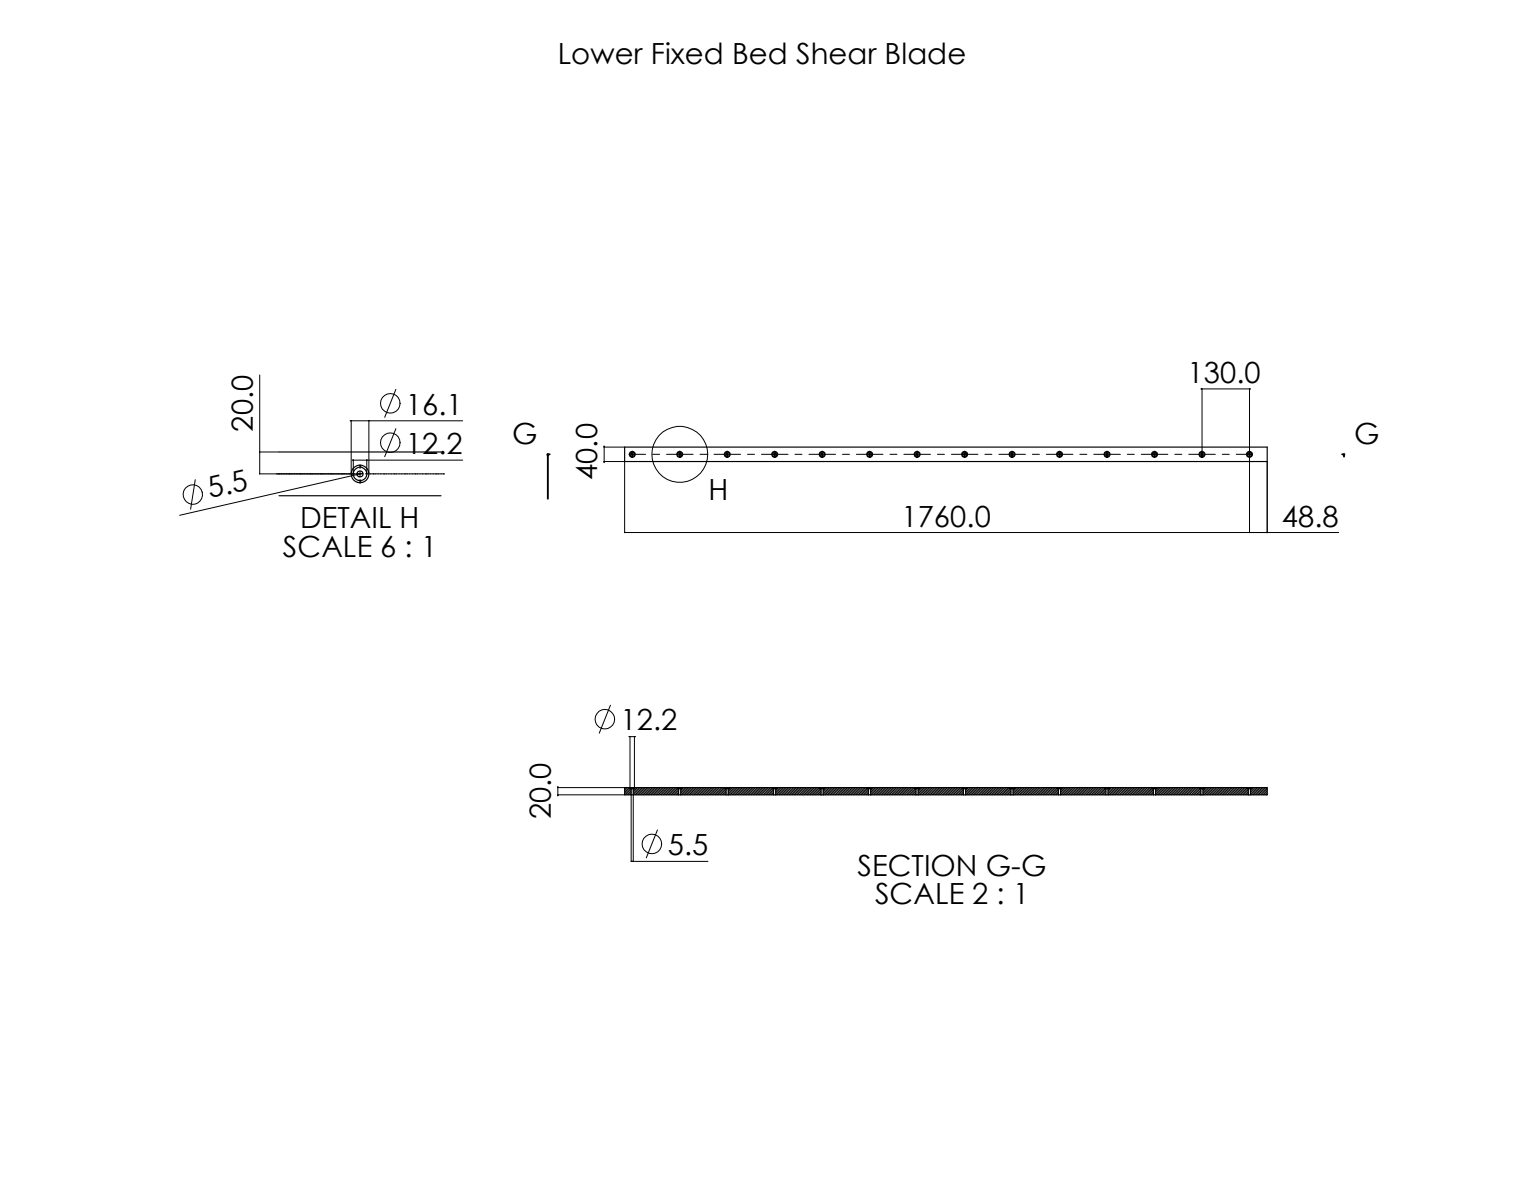
ISO-10303-21;
HEADER;
FILE_DESCRIPTION (('STEP AP214'),
    '1' );
FILE_NAME ('Lower Fixed Bed Shear Blade.step',
    '2026-10-21T17:07:05',
    ( '' ),
    ( '' ),
    'SwSTEP 2.0',
    'SolidWorks 2025',
    '' );
FILE_SCHEMA (( 'AUTOMOTIVE_DESIGN' ));
ENDSEC;

DATA;
#64=DIRECTION ( 'NONE',  ( 0.000000000000000000, 0.000000000000000000, 1.000000000000000000 ) ) ;
#90=EDGE_CURVE ( 'NONE', #25509, #42507, #33534, .T. ) ;
#102=FACE_OUTER_BOUND ( 'NONE', #34490, .T. ) ;
#109=EDGE_CURVE ( 'NONE', #28297, #10740, #37704, .T. ) ;
#136=CARTESIAN_POINT ( 'NONE',  ( 701.1634899080286232, 259.9999999999999432, -208.0249999999989825 ) ) ;
#150=CARTESIAN_POINT ( 'NONE',  ( 441.1634899080286232, 259.9999999999999432, -208.0249999999972488 ) ) ;
#156=CARTESIAN_POINT ( 'NONE',  ( 311.1634899080286232, 260.0000000000000000, -208.0249999999963109 ) ) ;
#168=CARTESIAN_POINT ( 'NONE',  ( -338.8365100919713200, 256.5000000000001137, -199.9999999999917861 ) ) ;
#175=ORIENTED_EDGE ( 'NONE', *, *, #22188, .T. ) ;
#215=DIRECTION ( 'NONE',  ( 0.000000000000000000, 0.000000000000000000, 1.000000000000000000 ) ) ;
#249=DIRECTION ( 'NONE',  ( -0.000000000000000000, 1.000000000000000000, -0.000000000000000000 ) ) ;
#252=ORIENTED_EDGE ( 'NONE', *, *, #2953, .T. ) ;
#299=ORIENTED_EDGE ( 'NONE', *, *, #28143, .F. ) ;
#323=CIRCLE ( 'NONE', #21716, 6.118999999999985562 ) ;
#329=AXIS2_PLACEMENT_3D ( 'NONE', #6576, #23655, #31056 ) ;
#334=PLANE ( 'NONE',  #18115 ) ;
#335=DIRECTION ( 'NONE',  ( -0.000000000000000000, 1.000000000000000000, -0.000000000000000000 ) ) ;
#344=CARTESIAN_POINT ( 'NONE',  ( 181.1634899080285948, 256.5000000000000000, -202.7499999999952820 ) ) ;
#355=AXIS2_PLACEMENT_3D ( 'NONE', #23312, #5092, #16163 ) ;
#363=DIRECTION ( 'NONE',  ( 0.000000000000000000, 0.000000000000000000, 1.000000000000000000 ) ) ;
#364=CARTESIAN_POINT ( 'NONE',  ( -202.7175100919714055, 256.5000000000001137, -199.9999999999926956 ) ) ;
#373=DIRECTION ( 'NONE',  ( 0.000000000000000000, 0.000000000000000000, 1.000000000000000000 ) ) ;
#391=CYLINDRICAL_SURFACE ( 'NONE', #1235, 2.749999999999863665 ) ;
#409=EDGE_CURVE ( 'NONE', #40245, #10694, #7775, .T. ) ;
#413=ORIENTED_EDGE ( 'NONE', *, *, #14771, .T. ) ;
#431=EDGE_CURVE ( 'NONE', #22786, #36028, #26937, .T. ) ;
#433=CARTESIAN_POINT ( 'NONE',  ( -78.83651009197140525, 240.0000000000000568, -199.9999999999936051 ) ) ;
#438=ORIENTED_EDGE ( 'NONE', *, *, #28628, .T. ) ;
#442=CARTESIAN_POINT ( 'NONE',  ( -852.7175100919713486, 256.5000000000002274, -199.9999999999881481 ) ) ;
#446=DIRECTION ( 'NONE',  ( -0.000000000000000000, 1.000000000000000000, -0.000000000000000000 ) ) ;
#448=VECTOR ( 'NONE', #36830, 999.9999999999998863 ) ;
#457=ADVANCED_FACE ( 'NONE', ( #28210 ), #41866, .F. ) ;
#466=VECTOR ( 'NONE', #30929, 1000.000000000000000 ) ;
#470=CARTESIAN_POINT ( 'NONE',  ( 831.1634899080286232, 259.9999999999998863, -199.9999999999999432 ) ) ;
#485=DIRECTION ( 'NONE',  ( -0.000000000000000000, 1.000000000000000000, -0.000000000000000000 ) ) ;
#490=AXIS2_PLACEMENT_3D ( 'NONE', #32758, #32530, #29065 ) ;
#509=DIRECTION ( 'NONE',  ( 0.000000000000000000, -1.000000000000000000, 0.000000000000000000 ) ) ;
#516=VECTOR ( 'NONE', #12520, 1000.000000000000000 ) ;
#521=EDGE_CURVE ( 'NONE', #12460, #20164, #17350, .T. ) ;
#527=ORIENTED_EDGE ( 'NONE', *, *, #24678, .F. ) ;
#530=ORIENTED_EDGE ( 'NONE', *, *, #3202, .F. ) ;
#547=CARTESIAN_POINT ( 'NONE',  ( 311.1634899080286232, 260.0000000000000000, -199.9999999999963336 ) ) ;
#567=CARTESIAN_POINT ( 'NONE',  ( 441.1634899080286232, 256.4999999999999432, -206.1189999999972144 ) ) ;
#569=EDGE_CURVE ( 'NONE', #23226, #12347, #33564, .T. ) ;
#599=LINE ( 'NONE', #35460, #21044 ) ;
#622=ADVANCED_FACE ( 'NONE', ( #10912, #13916, #35146, #24509, #31678, #3282, #39091, #20817, #34470, #34916, #6977, #31002, #31460, #31226, #3523 ), #24054, .F. ) ;
#663=CARTESIAN_POINT ( 'NONE',  ( -208.8365100919714052, 256.5000000000001137, -206.1189999999926954 ) ) ;
#664=DIRECTION ( 'NONE',  ( -0.000000000000000000, 1.000000000000000000, -0.000000000000000000 ) ) ;
#668=ORIENTED_EDGE ( 'NONE', *, *, #5793, .T. ) ;
#675=ADVANCED_FACE ( 'NONE', ( #20599 ), #14394, .F. ) ;
#678=CARTESIAN_POINT ( 'NONE',  ( 441.1634899080286232, 259.9999999999999432, -199.9999999999972431 ) ) ;
#682=DIRECTION ( 'NONE',  ( -0.000000000000000000, 1.000000000000000000, -0.000000000000000000 ) ) ;
#701=ORIENTED_EDGE ( 'NONE', *, *, #28035, .F. ) ;
#714=CARTESIAN_POINT ( 'NONE',  ( -78.83651009197140525, 256.5000000000000568, -202.7499999999934914 ) ) ;
#715=EDGE_CURVE ( 'NONE', #2952, #17860, #21035, .T. ) ;
#724=CARTESIAN_POINT ( 'NONE',  ( 571.1634899080285095, 259.9999999999999432, -199.9999999999981526 ) ) ;
#731=CARTESIAN_POINT ( 'NONE',  ( -208.8365100919714052, 258.0940000000001078, -193.8809999999926674 ) ) ;
#733=DIRECTION ( 'NONE',  ( -0.000000000000000000, 1.000000000000000000, -0.000000000000000000 ) ) ;
#746=ADVANCED_FACE ( 'NONE', ( #35841, #28910 ), #15052, .F. ) ;
#773=DIRECTION ( 'NONE',  ( 0.000000000000000000, 0.000000000000000000, 1.000000000000000000 ) ) ;
#774=ORIENTED_EDGE ( 'NONE', *, *, #715, .T. ) ;
#827=FACE_OUTER_BOUND ( 'NONE', #26973, .T. ) ;
#832=FACE_BOUND ( 'NONE', #35157, .T. ) ;
#873=CARTESIAN_POINT ( 'NONE',  ( -728.8365100919714905, 240.0000000000001990, -199.9999999999890861 ) ) ;
#891=DIRECTION ( 'NONE',  ( 0.000000000000000000, 0.000000000000000000, 1.000000000000000000 ) ) ;
#895=DIRECTION ( 'NONE',  ( 0.000000000000000000, 0.000000000000000000, 1.000000000000000000 ) ) ;
#910=DIRECTION ( 'NONE',  ( -0.000000000000000000, 1.000000000000000000, -0.000000000000000000 ) ) ;
#919=EDGE_CURVE ( 'NONE', #14904, #3234, #12181, .T. ) ;
#958=ORIENTED_EDGE ( 'NONE', *, *, #40695, .F. ) ;
#970=ADVANCED_FACE ( 'NONE', ( #44230 ), #9588, .F. ) ;
#973=ORIENTED_EDGE ( 'NONE', *, *, #27496, .F. ) ;
#980=AXIS2_PLACEMENT_3D ( 'NONE', #10116, #31353, #10336 ) ;
#996=CARTESIAN_POINT ( 'NONE',  ( -728.8365100919714905, 240.0000000000001990, -199.9999999999890861 ) ) ;
#1006=DIRECTION ( 'NONE',  ( -0.000000000000000000, 1.000000000000000000, -0.000000000000000000 ) ) ;
#1009=EDGE_CURVE ( 'NONE', #13600, #26360, #44455, .T. ) ;
#1018=ORIENTED_EDGE ( 'NONE', *, *, #15333, .T. ) ;
#1019=EDGE_CURVE ( 'NONE', #16583, #8247, #41590, .T. ) ;
#1047=CIRCLE ( 'NONE', #22428, 8.024999999999948841 ) ;
#1051=FACE_OUTER_BOUND ( 'NONE', #38699, .T. ) ;
#1054=FACE_BOUND ( 'NONE', #24359, .T. ) ;
#1074=ORIENTED_EDGE ( 'NONE', *, *, #6356, .T. ) ;
#1088=ORIENTED_EDGE ( 'NONE', *, *, #17337, .F. ) ;
#1099=CARTESIAN_POINT ( 'NONE',  ( 181.1634899080285948, 260.0000000000000000, -199.9999999999953957 ) ) ;
#1102=ORIENTED_EDGE ( 'NONE', *, *, #32866, .T. ) ;
#1119=CONICAL_SURFACE ( 'NONE', #17339, 8.024999999999948841, 0.7853981633974337351 ) ;
#1129=AXIS2_PLACEMENT_3D ( 'NONE', #37239, #8853, #9534 ) ;
#1134=CARTESIAN_POINT ( 'NONE',  ( 51.16348990802859475, 260.0000000000000568, -199.9999999999945146 ) ) ;
#1143=AXIS2_PLACEMENT_3D ( 'NONE', #37634, #44811, #30468 ) ;
#1174=AXIS2_PLACEMENT_3D ( 'NONE', #4069, #8002, #22282 ) ;
#1178=VECTOR ( 'NONE', #33127, 1000.000000000000114 ) ;
#1180=CARTESIAN_POINT ( 'NONE',  ( -468.8365100919714337, 256.5000000000001705, -202.7499999999907914 ) ) ;
#1201=ORIENTED_EDGE ( 'NONE', *, *, #10607, .T. ) ;
#1218=CARTESIAN_POINT ( 'NONE',  ( -728.8365100919714905, 260.0000000000001705, -199.9999999999890861 ) ) ;
#1235=AXIS2_PLACEMENT_3D ( 'NONE', #25558, #24866, #4321 ) ;
#1239=EDGE_CURVE ( 'NONE', #18073, #20679, #43780, .T. ) ;
#1246=VECTOR ( 'NONE', #42062, 1000.000000000000000 ) ;
#1251=ORIENTED_EDGE ( 'NONE', *, *, #3202, .T. ) ;
#1252=AXIS2_PLACEMENT_3D ( 'NONE', #35298, #45241, #3675 ) ;
#1269=ORIENTED_EDGE ( 'NONE', *, *, #27496, .T. ) ;
#1275=FACE_BOUND ( 'NONE', #36919, .T. ) ;
#1284=EDGE_CURVE ( 'NONE', #36701, #8042, #25367, .T. ) ;
#1288=CYLINDRICAL_SURFACE ( 'NONE', #20808, 2.749999999999863665 ) ;
#1322=ORIENTED_EDGE ( 'NONE', *, *, #35586, .F. ) ;
#1338=ADVANCED_FACE ( 'NONE', ( #17665 ), #34740, .F. ) ;
#1345=EDGE_LOOP ( 'NONE', ( #527, #16375 ) ) ;
#1364=DIRECTION ( 'NONE',  ( -0.000000000000000000, 1.000000000000000000, -0.000000000000000000 ) ) ;
#1383=ORIENTED_EDGE ( 'NONE', *, *, #22701, .F. ) ;
#1387=DIRECTION ( 'NONE',  ( -0.000000000000000000, 1.000000000000000000, -0.000000000000000000 ) ) ;
#1406=DIRECTION ( 'NONE',  ( 8.659560562354932858E-17, 0.7071067811865474617, -0.7071067811865474617 ) ) ;
#1432=ORIENTED_EDGE ( 'NONE', *, *, #25271, .T. ) ;
#1437=DIRECTION ( 'NONE',  ( 0.000000000000000000, 0.000000000000000000, 1.000000000000000000 ) ) ;
#1458=ORIENTED_EDGE ( 'NONE', *, *, #12287, .F. ) ;
#1471=ORIENTED_EDGE ( 'NONE', *, *, #8622, .T. ) ;
#1473=EDGE_LOOP ( 'NONE', ( #35327, #6545 ) ) ;
#1486=CARTESIAN_POINT ( 'NONE',  ( 441.1634899080286232, 259.9999999999999432, -199.9999999999972431 ) ) ;
#1521=EDGE_LOOP ( 'NONE', ( #973, #3985, #6124, #36419 ) ) ;
#1527=ORIENTED_EDGE ( 'NONE', *, *, #24375, .F. ) ;
#1572=ORIENTED_EDGE ( 'NONE', *, *, #41017, .T. ) ;
#1575=CYLINDRICAL_SURFACE ( 'NONE', #28444, 2.749999999999835687 ) ;
#1578=EDGE_CURVE ( 'NONE', #27745, #12435, #3971, .T. ) ;
#1584=DIRECTION ( 'NONE',  ( 0.000000000000000000, -1.000000000000000000, 0.000000000000000000 ) ) ;
#1614=DIRECTION ( 'NONE',  ( 0.000000000000000000, 0.000000000000000000, 1.000000000000000000 ) ) ;
#1671=DIRECTION ( 'NONE',  ( 1.892425610156518354E-16, 1.000000000000000000, -0.000000000000000000 ) ) ;
#1687=ORIENTED_EDGE ( 'NONE', *, *, #6335, .T. ) ;
#1730=CARTESIAN_POINT ( 'NONE',  ( 181.1634899080285948, 258.0939999999999941, -199.9999999999953957 ) ) ;
#1737=AXIS2_PLACEMENT_3D ( 'NONE', #29256, #18625, #39664 ) ;
#1789=EDGE_CURVE ( 'NONE', #18281, #21321, #6935, .T. ) ;
#1792=CARTESIAN_POINT ( 'NONE',  ( 181.1634899080285948, 258.0939999999999941, -193.8809999999953959 ) ) ;
#1821=DIRECTION ( 'NONE',  ( 8.659560562354884787E-17, 0.7071067811865513475, -0.7071067811865435759 ) ) ;
#1837=AXIS2_PLACEMENT_3D ( 'NONE', #10668, #24752, #17142 ) ;
#1841=AXIS2_PLACEMENT_3D ( 'NONE', #25140, #18248, #891 ) ;
#1848=EDGE_CURVE ( 'NONE', #24881, #7749, #17997, .T. ) ;
#1859=VECTOR ( 'NONE', #34701, 1000.000000000000000 ) ;
#1863=DIRECTION ( 'NONE',  ( 0.000000000000000000, 0.000000000000000000, 1.000000000000000000 ) ) ;
#1883=FACE_OUTER_BOUND ( 'NONE', #18472, .T. ) ;
#1903=CARTESIAN_POINT ( 'NONE',  ( 51.16348990802859475, 260.0000000000000568, -191.9749999999945089 ) ) ;
#1912=EDGE_LOOP ( 'NONE', ( #2855, #11798 ) ) ;
#1929=EDGE_LOOP ( 'NONE', ( #4719, #16342 ) ) ;
#1936=CARTESIAN_POINT ( 'NONE',  ( 571.1634899080285095, 259.9999999999999432, -191.9749999999982037 ) ) ;
#1953=AXIS2_PLACEMENT_3D ( 'NONE', #25021, #7703, #5081 ) ;
#1967=DIRECTION ( 'NONE',  ( -0.000000000000000000, 1.000000000000000000, -0.000000000000000000 ) ) ;
#1971=DIRECTION ( 'NONE',  ( 0.000000000000000000, 0.000000000000000000, 1.000000000000000000 ) ) ;
#2015=DIRECTION ( 'NONE',  ( 1.892425610156518354E-16, 1.000000000000000000, -0.000000000000000000 ) ) ;
#2021=ORIENTED_EDGE ( 'NONE', *, *, #18268, .F. ) ;
#2032=LINE ( 'NONE', #16126, #38083 ) ;
#2040=FACE_OUTER_BOUND ( 'NONE', #4448, .T. ) ;
#2052=ORIENTED_EDGE ( 'NONE', *, *, #41702, .T. ) ;
#2060=CARTESIAN_POINT ( 'NONE',  ( 51.16348990802859475, 260.0000000000000568, -208.0249999999945203 ) ) ;
#2071=DIRECTION ( 'NONE',  ( -0.000000000000000000, 1.000000000000000000, -0.000000000000000000 ) ) ;
#2089=DIRECTION ( 'NONE',  ( -1.000000000000000000, 0.000000000000000000, 0.000000000000000000 ) ) ;
#2109=ORIENTED_EDGE ( 'NONE', *, *, #27219, .T. ) ;
#2117=EDGE_CURVE ( 'NONE', #32983, #10586, #6970, .T. ) ;
#2155=AXIS2_PLACEMENT_3D ( 'NONE', #9924, #17090, #45047 ) ;
#2174=FACE_OUTER_BOUND ( 'NONE', #8874, .T. ) ;
#2183=DIRECTION ( 'NONE',  ( 0.000000000000000000, 0.000000000000000000, 1.000000000000000000 ) ) ;
#2184=DIRECTION ( 'NONE',  ( 0.000000000000000000, 0.000000000000000000, 1.000000000000000000 ) ) ;
#2187=DIRECTION ( 'NONE',  ( 1.892425610156518354E-16, 1.000000000000000000, -0.000000000000000000 ) ) ;
#2204=VERTEX_POINT ( 'NONE', #42077 ) ;
#2318=EDGE_LOOP ( 'NONE', ( #31488, #3719, #20337, #11430 ) ) ;
#2344=AXIS2_PLACEMENT_3D ( 'NONE', #37289, #19743, #2183 ) ;
#2350=DIRECTION ( 'NONE',  ( -0.000000000000000000, 1.000000000000000000, -0.000000000000000000 ) ) ;
#2371=AXIS2_PLACEMENT_3D ( 'NONE', #8273, #12193, #22338 ) ;
#2376=ORIENTED_EDGE ( 'NONE', *, *, #18681, .F. ) ;
#2429=ORIENTED_EDGE ( 'NONE', *, *, #24599, .T. ) ;
#2436=ORIENTED_EDGE ( 'NONE', *, *, #569, .F. ) ;
#2452=CYLINDRICAL_SURFACE ( 'NONE', #33609, 2.749999999999835687 ) ;
#2458=CIRCLE ( 'NONE', #980, 2.749999999999919176 ) ;
#2459=CARTESIAN_POINT ( 'NONE',  ( -598.8365100919716042, 256.5000000000001705, -193.8809999999899674 ) ) ;
#2469=CYLINDRICAL_SURFACE ( 'NONE', #21640, 2.749999999999835687 ) ;
#2489=ORIENTED_EDGE ( 'NONE', *, *, #9146, .F. ) ;
#2496=ORIENTED_EDGE ( 'NONE', *, *, #15984, .F. ) ;
#2521=VECTOR ( 'NONE', #28121, 1000.000000000000000 ) ;
#2523=CARTESIAN_POINT ( 'NONE',  ( -858.8365100919713768, 260.0000000000002274, -202.7499999999880345 ) ) ;
#2534=CARTESIAN_POINT ( 'NONE',  ( 571.1634899080285095, 256.4999999999999432, -199.9999999999981526 ) ) ;
#2538=VECTOR ( 'NONE', #9306, 1000.000000000000114 ) ;
#2565=VERTEX_POINT ( 'NONE', #39304 ) ;
#2570=AXIS2_PLACEMENT_3D ( 'NONE', #24286, #41626, #38393 ) ;
#2573=EDGE_LOOP ( 'NONE', ( #31065, #5375, #41524, #11084 ) ) ;
#2578=CIRCLE ( 'NONE', #34293, 2.749999999999842792 ) ;
#2586=VECTOR ( 'NONE', #42191, 1000.000000000000000 ) ;
#2621=EDGE_LOOP ( 'NONE', ( #6438, #44076, #22778, #12903 ) ) ;
#2629=AXIS2_PLACEMENT_3D ( 'NONE', #21604, #35686, #25291 ) ;
#2650=CARTESIAN_POINT ( 'NONE',  ( -338.8365100919713200, 240.0000000000001137, -199.9999999999917861 ) ) ;
#2665=DIRECTION ( 'NONE',  ( 0.000000000000000000, -1.000000000000000000, 0.000000000000000000 ) ) ;
#2691=AXIS2_PLACEMENT_3D ( 'NONE', #6556, #20411, #34260 ) ;
#2695=ADVANCED_FACE ( 'NONE', ( #18302 ), #32380, .F. ) ;
#2701=LINE ( 'NONE', #16798, #7052 ) ;
#2704=CARTESIAN_POINT ( 'NONE',  ( 571.1634899080285095, 256.4999999999999432, -199.9999999999981526 ) ) ;
#2718=MANIFOLD_SOLID_BREP ( 'CBORE for M5 Hex Head Bolt1[2]', #11423 ) ;
#2728=ORIENTED_EDGE ( 'NONE', *, *, #6661, .F. ) ;
#2736=VERTEX_POINT ( 'NONE', #44578 ) ;
#2744=EDGE_CURVE ( 'NONE', #13947, #12019, #37222, .T. ) ;
#2755=CARTESIAN_POINT ( 'NONE',  ( -879.9999999999992042, 260.0000000000002274, -219.9999999999999716 ) ) ;
#2758=CARTESIAN_POINT ( 'NONE',  ( -468.8365100919714337, 256.5000000000001705, -193.8809999999909053 ) ) ;
#2759=EDGE_CURVE ( 'NONE', #17388, #33219, #5502, .T. ) ;
#2800=AXIS2_PLACEMENT_3D ( 'NONE', #39327, #7928, #21531 ) ;
#2822=CARTESIAN_POINT ( 'NONE',  ( -858.8365100919713768, 256.5000000000002274, -193.8809999999881768 ) ) ;
#2855=ORIENTED_EDGE ( 'NONE', *, *, #19344, .F. ) ;
#2860=DIRECTION ( 'NONE',  ( -0.000000000000000000, 1.000000000000000000, -0.000000000000000000 ) ) ;
#2874=LINE ( 'NONE', #13736, #20844 ) ;
#2894=PLANE ( 'NONE',  #39520 ) ;
#2930=EDGE_CURVE ( 'NONE', #29766, #7990, #23958, .T. ) ;
#2941=CARTESIAN_POINT ( 'NONE',  ( -879.9999999999992042, 260.0000000000002274, -179.9999999999999716 ) ) ;
#2952=VERTEX_POINT ( 'NONE', #44343 ) ;
#2953=EDGE_CURVE ( 'NONE', #7990, #29766, #45355, .T. ) ;
#2963=ORIENTED_EDGE ( 'NONE', *, *, #31104, .T. ) ;
#2980=EDGE_CURVE ( 'NONE', #44849, #11829, #23929, .T. ) ;
#3007=EDGE_CURVE ( 'NONE', #41246, #7001, #8498, .T. ) ;
#3035=EDGE_LOOP ( 'NONE', ( #21215, #32230 ) ) ;
#3037=DIRECTION ( 'NONE',  ( -0.000000000000000000, 1.000000000000000000, -0.000000000000000000 ) ) ;
#3044=LINE ( 'NONE', #38609, #24699 ) ;
#3052=DIRECTION ( 'NONE',  ( 0.000000000000000000, 0.000000000000000000, 1.000000000000000000 ) ) ;
#3068=DIRECTION ( 'NONE',  ( -1.000000000000000000, 0.000000000000000000, 0.000000000000000000 ) ) ;
#3137=CARTESIAN_POINT ( 'NONE',  ( -208.8365100919714052, 256.5000000000001137, -202.7499999999925819 ) ) ;
#3138=LINE ( 'NONE', #38714, #14438 ) ;
#3140=VERTEX_POINT ( 'NONE', #17553 ) ;
#3161=CARTESIAN_POINT ( 'NONE',  ( -468.8365100919714337, 240.0000000000001421, -202.7499999999907345 ) ) ;
#3182=DIRECTION ( 'NONE',  ( -1.000000000000000000, 1.892425610156518354E-16, -0.000000000000000000 ) ) ;
#3202=EDGE_CURVE ( 'NONE', #30680, #28948, #34290, .T. ) ;
#3205=VERTEX_POINT ( 'NONE', #45260 ) ;
#3234=VERTEX_POINT ( 'NONE', #24684 ) ;
#3282=FACE_BOUND ( 'NONE', #18764, .T. ) ;
#3290=CIRCLE ( 'NONE', #45331, 8.024999999999948841 ) ;
#3299=ORIENTED_EDGE ( 'NONE', *, *, #19907, .F. ) ;
#3302=ORIENTED_EDGE ( 'NONE', *, *, #40695, .T. ) ;
#3305=( NAMED_UNIT ( * ) PLANE_ANGLE_UNIT ( ) SI_UNIT ( $, .RADIAN. ) );
#3318=DIRECTION ( 'NONE',  ( -0.000000000000000000, 1.000000000000000000, -0.000000000000000000 ) ) ;
#3323=DIRECTION ( 'NONE',  ( 0.000000000000000000, 0.000000000000000000, 1.000000000000000000 ) ) ;
#3327=CIRCLE ( 'NONE', #20980, 6.118999999999985562 ) ;
#3329=VECTOR ( 'NONE', #38752, 999.9999999999998863 ) ;
#3334=CARTESIAN_POINT ( 'NONE',  ( -728.8365100919714905, 260.0000000000001705, -208.0249999999890349 ) ) ;
#3336=CIRCLE ( 'NONE', #30589, 2.749999999999919176 ) ;
#3352=AXIS2_PLACEMENT_3D ( 'NONE', #10849, #17778, #32078 ) ;
#3356=DIRECTION ( 'NONE',  ( 0.000000000000000000, 0.000000000000000000, 1.000000000000000000 ) ) ;
#3357=CARTESIAN_POINT ( 'NONE',  ( -722.7175100919714623, 256.5000000000001705, -199.9999999999890861 ) ) ;
#3373=AXIS2_PLACEMENT_3D ( 'NONE', #20882, #23659, #3356 ) ;
#3388=EDGE_CURVE ( 'NONE', #10815, #22607, #39504, .T. ) ;
#3391=VECTOR ( 'NONE', #32469, 999.9999999999998863 ) ;
#3439=EDGE_LOOP ( 'NONE', ( #17422, #16149, #26248, #25911 ) ) ;
#3441=CARTESIAN_POINT ( 'NONE',  ( 831.1634899080286232, 256.4999999999998863, -197.2500000000000284 ) ) ;
#3443=CARTESIAN_POINT ( 'NONE',  ( -858.8365100919713768, 258.0940000000002215, -193.8809999999881768 ) ) ;
#3461=CIRCLE ( 'NONE', #25583, 6.118999999999985562 ) ;
#3488=EDGE_CURVE ( 'NONE', #26915, #40829, #16634, .T. ) ;
#3494=EDGE_LOOP ( 'NONE', ( #1018, #39594 ) ) ;
#3500=AXIS2_PLACEMENT_3D ( 'NONE', #44971, #38722, #41966 ) ;
#3510=ADVANCED_FACE ( 'NONE', ( #3911 ), #28380, .F. ) ;
#3523=FACE_OUTER_BOUND ( 'NONE', #33807, .T. ) ;
#3549=EDGE_CURVE ( 'NONE', #39281, #38048, #37255, .T. ) ;
#3560=CARTESIAN_POINT ( 'NONE',  ( -598.8365100919716042, 260.0000000000001705, -199.9999999999899671 ) ) ;
#3562=ORIENTED_EDGE ( 'NONE', *, *, #17880, .T. ) ;
#3569=AXIS2_PLACEMENT_3D ( 'NONE', #27047, #27953, #42049 ) ;
#3586=CARTESIAN_POINT ( 'NONE',  ( 701.1634899080286232, 259.9999999999999432, -199.9999999999990337 ) ) ;
#3617=FACE_OUTER_BOUND ( 'NONE', #40533, .T. ) ;
#3636=VECTOR ( 'NONE', #9011, 1000.000000000000114 ) ;
#3659=ORIENTED_EDGE ( 'NONE', *, *, #40850, .T. ) ;
#3662=EDGE_LOOP ( 'NONE', ( #22676, #3827, #31750, #2963 ) ) ;
#3675=DIRECTION ( 'NONE',  ( -1.000000000000000000, 0.000000000000000000, 0.000000000000000000 ) ) ;
#3679=CARTESIAN_POINT ( 'NONE',  ( -728.8365100919714905, 260.0000000000001705, -206.1189999999890574 ) ) ;
#3719=ORIENTED_EDGE ( 'NONE', *, *, #24375, .T. ) ;
#3721=DIRECTION ( 'NONE',  ( -0.000000000000000000, 1.000000000000000000, -0.000000000000000000 ) ) ;
#3774=DIRECTION ( 'NONE',  ( 0.000000000000000000, 0.000000000000000000, 1.000000000000000000 ) ) ;
#3775=CYLINDRICAL_SURFACE ( 'NONE', #33686, 2.749999999999863665 ) ;
#3787=DIRECTION ( 'NONE',  ( 0.000000000000000000, -0.000000000000000000, -1.000000000000000000 ) ) ;
#3827=ORIENTED_EDGE ( 'NONE', *, *, #13072, .F. ) ;
#3833=DIRECTION ( 'NONE',  ( 0.000000000000000000, 0.000000000000000000, 1.000000000000000000 ) ) ;
#3841=CARTESIAN_POINT ( 'NONE',  ( 51.16348990802859475, 260.0000000000000568, -199.9999999999945146 ) ) ;
#3842=EDGE_CURVE ( 'NONE', #40829, #26915, #24728, .T. ) ;
#3844=CYLINDRICAL_SURFACE ( 'NONE', #12912, 6.118999999999985562 ) ;
#3847=CARTESIAN_POINT ( 'NONE',  ( -858.8365100919713768, 256.5000000000002274, -199.9999999999881481 ) ) ;
#3858=ADVANCED_FACE ( 'NONE', ( #28917 ), #29596, .F. ) ;
#3862=CIRCLE ( 'NONE', #2344, 6.118999999999985562 ) ;
#3898=FACE_OUTER_BOUND ( 'NONE', #20408, .T. ) ;
#3905=FACE_BOUND ( 'NONE', #1345, .T. ) ;
#3911=FACE_OUTER_BOUND ( 'NONE', #37370, .T. ) ;
#3948=EDGE_LOOP ( 'NONE', ( #23305, #31638 ) ) ;
#3971=CIRCLE ( 'NONE', #15055, 2.749999999999919176 ) ;
#3978=ORIENTED_EDGE ( 'NONE', *, *, #6649, .F. ) ;
#3985=ORIENTED_EDGE ( 'NONE', *, *, #37858, .F. ) ;
#3992=ORIENTED_EDGE ( 'NONE', *, *, #37651, .F. ) ;
#4002=ORIENTED_EDGE ( 'NONE', *, *, #13445, .T. ) ;
#4007=ORIENTED_EDGE ( 'NONE', *, *, #13993, .F. ) ;
#4033=CARTESIAN_POINT ( 'NONE',  ( 879.9999999999992042, 259.9999999999998863, -219.9999999999999716 ) ) ;
#4052=EDGE_CURVE ( 'NONE', #40519, #28937, #18128, .T. ) ;
#4058=CIRCLE ( 'NONE', #19533, 2.749999999999919176 ) ;
#4062=CARTESIAN_POINT ( 'NONE',  ( 571.1634899080285095, 259.9999999999999432, -199.9999999999981526 ) ) ;
#4069=CARTESIAN_POINT ( 'NONE',  ( -468.8365100919714337, 256.5000000000001705, -199.9999999999908766 ) ) ;
#4087=CIRCLE ( 'NONE', #9970, 6.118999999999985562 ) ;
#4096=VECTOR ( 'NONE', #2071, 1000.000000000000000 ) ;
#4117=ORIENTED_EDGE ( 'NONE', *, *, #31446, .T. ) ;
#4128=EDGE_CURVE ( 'NONE', #29032, #40245, #25599, .T. ) ;
#4148=DIRECTION ( 'NONE',  ( 0.000000000000000000, -0.000000000000000000, -1.000000000000000000 ) ) ;
#4150=EDGE_CURVE ( 'NONE', #12347, #23226, #9248, .T. ) ;
#4168=AXIS2_PLACEMENT_3D ( 'NONE', #23038, #40839, #9199 ) ;
#4173=VECTOR ( 'NONE', #3721, 1000.000000000000000 ) ;
#4192=CARTESIAN_POINT ( 'NONE',  ( -728.8365100919714905, 240.0000000000001990, -197.2499999999891998 ) ) ;
#4216=DIRECTION ( 'NONE',  ( 0.000000000000000000, -0.000000000000000000, -1.000000000000000000 ) ) ;
#4237=ORIENTED_EDGE ( 'NONE', *, *, #5197, .T. ) ;
#4241=ORIENTED_EDGE ( 'NONE', *, *, #14801, .F. ) ;
#4249=CARTESIAN_POINT ( 'NONE',  ( 879.9999999999992042, 259.9999999999998863, -179.9999999999999716 ) ) ;
#4252=CARTESIAN_POINT ( 'NONE',  ( -858.8365100919713768, 260.0000000000002274, -199.9999999999881481 ) ) ;
#4276=DIRECTION ( 'NONE',  ( 0.000000000000000000, 0.000000000000000000, 1.000000000000000000 ) ) ;
#4302=CARTESIAN_POINT ( 'NONE',  ( 441.1634899080286232, 259.9999999999999432, -199.9999999999972431 ) ) ;
#4310=DIRECTION ( 'NONE',  ( 0.000000000000000000, 0.000000000000000000, 1.000000000000000000 ) ) ;
#4321=DIRECTION ( 'NONE',  ( 0.000000000000000000, 0.000000000000000000, 1.000000000000000000 ) ) ;
#4322=CARTESIAN_POINT ( 'NONE',  ( -468.8365100919714337, 256.5000000000001705, -206.1189999999908764 ) ) ;
#4328=DIRECTION ( 'NONE',  ( -0.000000000000000000, 1.000000000000000000, -0.000000000000000000 ) ) ;
#4338=ORIENTED_EDGE ( 'NONE', *, *, #32534, .F. ) ;
#4410=LINE ( 'NONE', #18501, #43969 ) ;
#4415=ORIENTED_EDGE ( 'NONE', *, *, #23048, .T. ) ;
#4423=DIRECTION ( 'NONE',  ( 8.659560562354807133E-17, 0.7071067811865578978, -0.7071067811865372477 ) ) ;
#4431=DIRECTION ( 'NONE',  ( -0.000000000000000000, 1.000000000000000000, -0.000000000000000000 ) ) ;
#4448=EDGE_LOOP ( 'NONE', ( #44211, #4584 ) ) ;
#4497=ORIENTED_EDGE ( 'NONE', *, *, #11378, .T. ) ;
#4510=VERTEX_POINT ( 'NONE', #4798 ) ;
#4524=CARTESIAN_POINT ( 'NONE',  ( 831.1634899080286232, 259.9999999999998863, -199.9999999999999432 ) ) ;
#4538=DIRECTION ( 'NONE',  ( -0.000000000000000000, 1.000000000000000000, -0.000000000000000000 ) ) ;
#4539=DIRECTION ( 'NONE',  ( -0.000000000000000000, 1.000000000000000000, -0.000000000000000000 ) ) ;
#4549=AXIS2_PLACEMENT_3D ( 'NONE', #35131, #31666, #20131 ) ;
#4555=ORIENTED_EDGE ( 'NONE', *, *, #16239, .T. ) ;
#4560=EDGE_LOOP ( 'NONE', ( #35172, #23960, #35397, #20708 ) ) ;
#4573=DIRECTION ( 'NONE',  ( -0.000000000000000000, 1.000000000000000000, -0.000000000000000000 ) ) ;
#4574=VERTEX_POINT ( 'NONE', #11956 ) ;
#4579=CARTESIAN_POINT ( 'NONE',  ( 441.1634899080286232, 259.9999999999999432, -191.9749999999972374 ) ) ;
#4584=ORIENTED_EDGE ( 'NONE', *, *, #17975, .T. ) ;
#4596=ORIENTED_EDGE ( 'NONE', *, *, #18756, .T. ) ;
#4600=CARTESIAN_POINT ( 'NONE',  ( -598.8365100919716042, 260.0000000000001705, -199.9999999999899671 ) ) ;
#4622=EDGE_CURVE ( 'NONE', #10881, #28279, #27703, .T. ) ;
#4629=VECTOR ( 'NONE', #39478, 1000.000000000000000 ) ;
#4662=DIRECTION ( 'NONE',  ( -0.000000000000000000, 1.000000000000000000, -0.000000000000000000 ) ) ;
#4663=ORIENTED_EDGE ( 'NONE', *, *, #37891, .T. ) ;
#4666=EDGE_CURVE ( 'NONE', #18328, #5387, #37183, .T. ) ;
#4670=ADVANCED_FACE ( 'NONE', ( #28490 ), #42807, .F. ) ;
#4707=DIRECTION ( 'NONE',  ( -0.000000000000000000, 1.000000000000000000, -0.000000000000000000 ) ) ;
#4719=ORIENTED_EDGE ( 'NONE', *, *, #26079, .F. ) ;
#4736=CARTESIAN_POINT ( 'NONE',  ( 441.1634899080286232, 259.9999999999999432, -199.9999999999972431 ) ) ;
#4744=DIRECTION ( 'NONE',  ( 0.000000000000000000, 0.000000000000000000, 1.000000000000000000 ) ) ;
#4748=CARTESIAN_POINT ( 'NONE',  ( 311.1634899080286232, 256.5000000000000000, -199.9999999999963336 ) ) ;
#4749=DIRECTION ( 'NONE',  ( 1.892425610156518354E-16, 1.000000000000000000, -0.000000000000000000 ) ) ;
#4760=CARTESIAN_POINT ( 'NONE',  ( -208.8365100919714052, 260.0000000000001137, -191.9749999999926899 ) ) ;
#4783=ORIENTED_EDGE ( 'NONE', *, *, #20154, .T. ) ;
#4797=AXIS2_PLACEMENT_3D ( 'NONE', #31895, #12938, #19635 ) ;
#4798=CARTESIAN_POINT ( 'NONE',  ( 571.1634899080285095, 256.4999999999999432, -202.7499999999980673 ) ) ;
#4816=AXIS2_PLACEMENT_3D ( 'NONE', #43754, #4978, #25975 ) ;
#4823=LINE ( 'NONE', #26048, #23213 ) ;
#4829=DIRECTION ( 'NONE',  ( 0.000000000000000000, 0.000000000000000000, 1.000000000000000000 ) ) ;
#4842=CIRCLE ( 'NONE', #2629, 8.025000000000003908 ) ;
#4845=APPLICATION_CONTEXT ( 'automotive_design' ) ;
#4865=CARTESIAN_POINT ( 'NONE',  ( 311.1634899080286232, 260.0000000000000000, -191.9749999999963279 ) ) ;
#4892=CARTESIAN_POINT ( 'NONE',  ( -78.83651009197140525, 240.0000000000000568, -199.9999999999936051 ) ) ;
#4909=DIRECTION ( 'NONE',  ( -1.000000000000000000, 0.000000000000000000, 0.000000000000000000 ) ) ;
#4910=DIRECTION ( 'NONE',  ( -0.000000000000000000, 1.000000000000000000, -0.000000000000000000 ) ) ;
#4917=CARTESIAN_POINT ( 'NONE',  ( 181.1634899080285948, 256.5000000000000000, -199.9999999999953957 ) ) ;
#4946=CIRCLE ( 'NONE', #1252, 2.749999999999863665 ) ;
#4947=ADVANCED_FACE ( 'NONE', ( #22451 ), #32643, .F. ) ;
#4968=DIRECTION ( 'NONE',  ( 0.000000000000000000, 0.7071067811865578978, 0.7071067811865372477 ) ) ;
#4971=PLANE ( 'NONE',  #8603 ) ;
#4978=DIRECTION ( 'NONE',  ( -0.000000000000000000, 1.000000000000000000, -0.000000000000000000 ) ) ;
#4981=CARTESIAN_POINT ( 'NONE',  ( 4.917854562272160638E-14, 260.0000000000000568, 0.000000000000000000 ) ) ;
#5042=VECTOR ( 'NONE', #10545, 1000.000000000000000 ) ;
#5052=CARTESIAN_POINT ( 'NONE',  ( 311.1634899080286232, 260.0000000000000000, -206.1189999999963050 ) ) ;
#5081=DIRECTION ( 'NONE',  ( 0.000000000000000000, 0.000000000000000000, 1.000000000000000000 ) ) ;
#5092=DIRECTION ( 'NONE',  ( -0.000000000000000000, 1.000000000000000000, -0.000000000000000000 ) ) ;
#5099=DIRECTION ( 'NONE',  ( 0.000000000000000000, 0.000000000000000000, 1.000000000000000000 ) ) ;
#5100=VECTOR ( 'NONE', #1406, 1000.000000000000114 ) ;
#5120=ORIENTED_EDGE ( 'NONE', *, *, #17979, .T. ) ;
#5128=EDGE_LOOP ( 'NONE', ( #31025, #26277, #29605, #7705 ) ) ;
#5155=CARTESIAN_POINT ( 'NONE',  ( -72.71751009197140547, 256.5000000000000568, -199.9999999999936051 ) ) ;
#5174=EDGE_LOOP ( 'NONE', ( #28986, #24546, #35045, #12721 ) ) ;
#5185=FACE_OUTER_BOUND ( 'NONE', #13079, .T. ) ;
#5191=DIRECTION ( 'NONE',  ( 0.000000000000000000, 0.000000000000000000, 1.000000000000000000 ) ) ;
#5194=FACE_BOUND ( 'NONE', #1912, .T. ) ;
#5197=EDGE_CURVE ( 'NONE', #44027, #33524, #21919, .T. ) ;
#5207=LINE ( 'NONE', #11707, #23915 ) ;
#5259=ORIENTED_EDGE ( 'NONE', *, *, #16521, .F. ) ;
#5280=EDGE_LOOP ( 'NONE', ( #30765, #27271, #4117, #12240 ) ) ;
#5298=VERTEX_POINT ( 'NONE', #12984 ) ;
#5311=CARTESIAN_POINT ( 'NONE',  ( 51.16348990802859475, 256.5000000000000568, -199.9999999999945146 ) ) ;
#5328=DIRECTION ( 'NONE',  ( -0.000000000000000000, 1.000000000000000000, -0.000000000000000000 ) ) ;
#5329=ORIENTED_EDGE ( 'NONE', *, *, #23218, .F. ) ;
#5346=DIRECTION ( 'NONE',  ( 0.000000000000000000, 0.000000000000000000, 1.000000000000000000 ) ) ;
#5347=CARTESIAN_POINT ( 'NONE',  ( 701.1634899080286232, 256.4999999999999432, -202.7499999999989484 ) ) ;
#5375=ORIENTED_EDGE ( 'NONE', *, *, #36816, .T. ) ;
#5383=VERTEX_POINT ( 'NONE', #5347 ) ;
#5387=VERTEX_POINT ( 'NONE', #40922 ) ;
#5410=EDGE_CURVE ( 'NONE', #26360, #5298, #6267, .T. ) ;
#5417=VECTOR ( 'NONE', #19310, 1000.000000000000000 ) ;
#5431=ADVANCED_FACE ( 'NONE', ( #1883 ), #20126, .F. ) ;
#5502=CIRCLE ( 'NONE', #32826, 6.119000000000013095 ) ;
#5549=CIRCLE ( 'NONE', #31374, 8.025000000000003908 ) ;
#5572=ORIENTED_EDGE ( 'NONE', *, *, #33916, .T. ) ;
#5580=AXIS2_PLACEMENT_3D ( 'NONE', #364, #36154, #21834 ) ;
#5582=FACE_OUTER_BOUND ( 'NONE', #12309, .T. ) ;
#5583=CARTESIAN_POINT ( 'NONE',  ( -338.8365100919713200, 260.0000000000001137, -199.9999999999917861 ) ) ;
#5589=CARTESIAN_POINT ( 'NONE',  ( -78.83651009197140525, 256.5000000000000568, -193.8809999999935769 ) ) ;
#5608=AXIS2_PLACEMENT_3D ( 'NONE', #20405, #2860, #45598 ) ;
#5613=AXIS2_PLACEMENT_3D ( 'NONE', #4302, #31997, #7762 ) ;
#5619=ORIENTED_EDGE ( 'NONE', *, *, #36478, .F. ) ;
#5621=AXIS2_PLACEMENT_3D ( 'NONE', #44533, #33682, #23273 ) ;
#5633=DIRECTION ( 'NONE',  ( -0.000000000000000000, 1.000000000000000000, -0.000000000000000000 ) ) ;
#5654=CIRCLE ( 'NONE', #490, 6.118999999999985562 ) ;
#5666=DIRECTION ( 'NONE',  ( 0.000000000000000000, 0.000000000000000000, 1.000000000000000000 ) ) ;
#5682=AXIS2_PLACEMENT_3D ( 'NONE', #26817, #30075, #9289 ) ;
#5689=EDGE_CURVE ( 'NONE', #2565, #32511, #24097, .T. ) ;
#5693=CIRCLE ( 'NONE', #14587, 6.118999999999985562 ) ;
#5700=DIRECTION ( 'NONE',  ( 0.000000000000000000, 0.000000000000000000, 1.000000000000000000 ) ) ;
#5714=EDGE_LOOP ( 'NONE', ( #28871, #23285, #1471, #25341 ) ) ;
#5757=ADVANCED_FACE ( 'NONE', ( #3905, #18000 ), #32070, .F. ) ;
#5761=ADVANCED_FACE ( 'NONE', ( #42925 ), #32540, .F. ) ;
#5764=ORIENTED_EDGE ( 'NONE', *, *, #17939, .F. ) ;
#5779=CARTESIAN_POINT ( 'NONE',  ( -598.8365100919716042, 258.0940000000001646, -199.9999999999899671 ) ) ;
#5793=EDGE_CURVE ( 'NONE', #8042, #36701, #13080, .T. ) ;
#5829=EDGE_CURVE ( 'NONE', #8740, #45067, #42592, .T. ) ;
#5888=CARTESIAN_POINT ( 'NONE',  ( 311.1634899080286232, 260.0000000000000000, -199.9999999999963336 ) ) ;
#5899=DIRECTION ( 'NONE',  ( -0.000000000000000000, 1.000000000000000000, -0.000000000000000000 ) ) ;
#5913=ORIENTED_EDGE ( 'NONE', *, *, #36558, .T. ) ;
#5920=LINE ( 'NONE', #40802, #26943 ) ;
#5971=ORIENTED_EDGE ( 'NONE', *, *, #43110, .F. ) ;
#5975=DIRECTION ( 'NONE',  ( -0.000000000000000000, 1.000000000000000000, -0.000000000000000000 ) ) ;
#6005=ORIENTED_EDGE ( 'NONE', *, *, #9679, .T. ) ;
#6014=LINE ( 'NONE', #16415, #10919 ) ;
#6020=EDGE_CURVE ( 'NONE', #14400, #22607, #32769, .T. ) ;
#6024=ORIENTED_EDGE ( 'NONE', *, *, #409, .T. ) ;
#6043=EDGE_CURVE ( 'NONE', #25919, #41246, #11529, .T. ) ;
#6059=LINE ( 'NONE', #13240, #1859 ) ;
#6075=DIRECTION ( 'NONE',  ( 1.000000000000000000, 0.000000000000000000, 0.000000000000000000 ) ) ;
#6089=DIRECTION ( 'NONE',  ( -0.000000000000000000, 1.000000000000000000, -0.000000000000000000 ) ) ;
#6092=CARTESIAN_POINT ( 'NONE',  ( 441.1634899080286232, 259.9999999999999432, -197.2499999999973852 ) ) ;
#6096=CARTESIAN_POINT ( 'NONE',  ( 831.1634899080286232, 259.9999999999998863, -199.9999999999999432 ) ) ;
#6120=EDGE_CURVE ( 'NONE', #28948, #42674, #8072, .T. ) ;
#6124=ORIENTED_EDGE ( 'NONE', *, *, #26419, .T. ) ;
#6145=DIRECTION ( 'NONE',  ( 0.000000000000000000, 0.000000000000000000, 1.000000000000000000 ) ) ;
#6153=CARTESIAN_POINT ( 'NONE',  ( -468.8365100919714337, 260.0000000000001705, -199.9999999999908766 ) ) ;
#6167=LINE ( 'NONE', #2941, #28653 ) ;
#6170=ORIENTED_EDGE ( 'NONE', *, *, #24477, .T. ) ;
#6267=LINE ( 'NONE', #30764, #516 ) ;
#6274=DIRECTION ( 'NONE',  ( -0.000000000000000000, 1.000000000000000000, -0.000000000000000000 ) ) ;
#6281=DIRECTION ( 'NONE',  ( 1.892425610156518354E-16, 1.000000000000000000, -0.000000000000000000 ) ) ;
#6288=CIRCLE ( 'NONE', #44636, 2.749999999999919176 ) ;
#6304=AXIS2_PLACEMENT_3D ( 'NONE', #873, #8267, #7828 ) ;
#6309=CIRCLE ( 'NONE', #32129, 2.749999999999919176 ) ;
#6323=FACE_OUTER_BOUND ( 'NONE', #17699, .T. ) ;
#6325=AXIS2_PLACEMENT_3D ( 'NONE', #14699, #17921, #363 ) ;
#6335=EDGE_CURVE ( 'NONE', #28948, #30680, #35859, .T. ) ;
#6343=DIRECTION ( 'NONE',  ( -0.000000000000000000, 1.000000000000000000, -0.000000000000000000 ) ) ;
#6353=CIRCLE ( 'NONE', #9935, 2.749999999999919176 ) ;
#6356=EDGE_CURVE ( 'NONE', #7990, #28297, #7271, .T. ) ;
#6357=FACE_OUTER_BOUND ( 'NONE', #38991, .T. ) ;
#6409=CYLINDRICAL_SURFACE ( 'NONE', #8359, 2.749999999999863665 ) ;
#6413=DIRECTION ( 'NONE',  ( -0.000000000000000000, 1.000000000000000000, -0.000000000000000000 ) ) ;
#6426=CIRCLE ( 'NONE', #36655, 2.749999999999835687 ) ;
#6436=CARTESIAN_POINT ( 'NONE',  ( -78.83651009197140525, 260.0000000000000568, -199.9999999999936051 ) ) ;
#6438=ORIENTED_EDGE ( 'NONE', *, *, #10590, .F. ) ;
#6506=CARTESIAN_POINT ( 'NONE',  ( 571.1634899080285095, 259.9999999999999432, -199.9999999999981526 ) ) ;
#6545=ORIENTED_EDGE ( 'NONE', *, *, #26084, .T. ) ;
#6556=CARTESIAN_POINT ( 'NONE',  ( 831.1634899080286232, 258.0939999999998804, -199.9999999999999432 ) ) ;
#6563=CARTESIAN_POINT ( 'NONE',  ( -208.8365100919714052, 260.0000000000001137, -199.9999999999926956 ) ) ;
#6576=CARTESIAN_POINT ( 'NONE',  ( -592.7175100919715760, 256.5000000000001705, -199.9999999999899671 ) ) ;
#6582=CARTESIAN_POINT ( 'NONE',  ( -858.8365100919713768, 256.5000000000002274, -202.7499999999880913 ) ) ;
#6583=FACE_OUTER_BOUND ( 'NONE', #27409, .T. ) ;
#6601=ORIENTED_EDGE ( 'NONE', *, *, #39633, .T. ) ;
#6649=EDGE_CURVE ( 'NONE', #20679, #40483, #8392, .T. ) ;
#6661=EDGE_CURVE ( 'NONE', #28937, #40519, #32165, .T. ) ;
#6698=ADVANCED_FACE ( 'NONE', ( #22461 ), #26260, .F. ) ;
#6706=CYLINDRICAL_SURFACE ( 'NONE', #3569, 6.118999999999985562 ) ;
#6742=DIRECTION ( 'NONE',  ( -0.000000000000000000, 1.000000000000000000, -0.000000000000000000 ) ) ;
#6770=ORIENTED_EDGE ( 'NONE', *, *, #17975, .F. ) ;
#6775=DIRECTION ( 'NONE',  ( -0.000000000000000000, 1.000000000000000000, -0.000000000000000000 ) ) ;
#6776=VERTEX_POINT ( 'NONE', #31948 ) ;
#6783=DIRECTION ( 'NONE',  ( -0.000000000000000000, 1.000000000000000000, -0.000000000000000000 ) ) ;
#6808=VERTEX_POINT ( 'NONE', #39829 ) ;
#6838=DIRECTION ( 'NONE',  ( -0.000000000000000000, 1.000000000000000000, -0.000000000000000000 ) ) ;
#6843=CARTESIAN_POINT ( 'NONE',  ( -879.9999999999992042, 260.0000000000002274, -219.9999999999999716 ) ) ;
#6859=LINE ( 'NONE', #34807, #3329 ) ;
#6861=ORIENTED_EDGE ( 'NONE', *, *, #44042, .T. ) ;
#6877=EDGE_LOOP ( 'NONE', ( #26194, #37083, #40389, #16437 ) ) ;
#6934=CARTESIAN_POINT ( 'NONE',  ( 831.1634899080286232, 239.9999999999998863, -202.7499999999998295 ) ) ;
#6935=CIRCLE ( 'NONE', #36445, 8.025000000000003908 ) ;
#6970=CIRCLE ( 'NONE', #34248, 2.749999999999835687 ) ;
#6977=FACE_BOUND ( 'NONE', #3494, .T. ) ;
#7001=VERTEX_POINT ( 'NONE', #9058 ) ;
#7018=AXIS2_PLACEMENT_3D ( 'NONE', #17935, #32004, #14477 ) ;
#7028=AXIS2_PLACEMENT_3D ( 'NONE', #19278, #29904, #43094 ) ;
#7033=DIRECTION ( 'NONE',  ( -0.000000000000000000, 1.000000000000000000, -0.000000000000000000 ) ) ;
#7041=AXIS2_PLACEMENT_3D ( 'NONE', #42304, #17833, #21063 ) ;
#7052=VECTOR ( 'NONE', #44972, 1000.000000000000000 ) ;
#7138=FACE_OUTER_BOUND ( 'NONE', #18912, .T. ) ;
#7146=ORIENTED_EDGE ( 'NONE', *, *, #14334, .T. ) ;
#7153=AXIS2_PLACEMENT_3D ( 'NONE', #17028, #31105, #13565 ) ;
#7167=CIRCLE ( 'NONE', #23358, 2.749999999999891642 ) ;
#7182=AXIS2_PLACEMENT_3D ( 'NONE', #28623, #31621, #42704 ) ;
#7193=LINE ( 'NONE', #35345, #4173 ) ;
#7196=DIRECTION ( 'NONE',  ( 0.000000000000000000, 0.7071067811865501263, 0.7071067811865449082 ) ) ;
#7197=EDGE_CURVE ( 'NONE', #40483, #21723, #6353, .T. ) ;
#7233=EDGE_LOOP ( 'NONE', ( #6601, #4596 ) ) ;
#7244=ORIENTED_EDGE ( 'NONE', *, *, #44042, .F. ) ;
#7265=DIRECTION ( 'NONE',  ( -0.000000000000000000, 1.000000000000000000, -0.000000000000000000 ) ) ;
#7271=LINE ( 'NONE', #31275, #25431 ) ;
#7285=DIRECTION ( 'NONE',  ( 0.000000000000000000, 0.000000000000000000, 1.000000000000000000 ) ) ;
#7289=ORIENTED_EDGE ( 'NONE', *, *, #5689, .T. ) ;
#7312=EDGE_LOOP ( 'NONE', ( #17467, #34606 ) ) ;
#7320=DIRECTION ( 'NONE',  ( 0.000000000000000000, 0.000000000000000000, 1.000000000000000000 ) ) ;
#7334=CARTESIAN_POINT ( 'NONE',  ( -728.8365100919714905, 260.0000000000001705, -199.9999999999890861 ) ) ;
#7352=AXIS2_PLACEMENT_3D ( 'NONE', #44672, #23628, #9568 ) ;
#7366=LINE ( 'NONE', #21217, #10792 ) ;
#7417=FACE_BOUND ( 'NONE', #11138, .T. ) ;
#7434=CARTESIAN_POINT ( 'NONE',  ( -468.8365100919714337, 260.0000000000001705, -199.9999999999908766 ) ) ;
#7456=ORIENTED_EDGE ( 'NONE', *, *, #3842, .T. ) ;
#7458=DIRECTION ( 'NONE',  ( -0.000000000000000000, 1.000000000000000000, -0.000000000000000000 ) ) ;
#7475=LINE ( 'NONE', #35627, #27014 ) ;
#7482=ORIENTED_EDGE ( 'NONE', *, *, #43367, .T. ) ;
#7489=DIRECTION ( 'NONE',  ( 0.000000000000000000, 0.000000000000000000, 1.000000000000000000 ) ) ;
#7492=CARTESIAN_POINT ( 'NONE',  ( -208.8365100919714052, 258.0940000000001078, -199.9999999999926956 ) ) ;
#7494=EDGE_CURVE ( 'NONE', #36773, #31071, #3044, .T. ) ;
#7505=DIRECTION ( 'NONE',  ( -1.000000000000000000, 1.880165489482579047E-16, 0.000000000000000000 ) ) ;
#7509=ORIENTED_EDGE ( 'NONE', *, *, #16501, .F. ) ;
#7523=ORIENTED_EDGE ( 'NONE', *, *, #23757, .F. ) ;
#7526=EDGE_LOOP ( 'NONE', ( #44778, #13250, #12647, #22491 ) ) ;
#7533=ORIENTED_EDGE ( 'NONE', *, *, #18143, .F. ) ;
#7550=EDGE_CURVE ( 'NONE', #10866, #11865, #2578, .T. ) ;
#7570=ORIENTED_EDGE ( 'NONE', *, *, #15389, .T. ) ;
#7627=VERTEX_POINT ( 'NONE', #2822 ) ;
#7640=LINE ( 'NONE', #8110, #14493 ) ;
#7644=ORIENTED_EDGE ( 'NONE', *, *, #43110, .T. ) ;
#7656=CARTESIAN_POINT ( 'NONE',  ( 181.1634899080285948, 260.0000000000000000, -191.9749999999953900 ) ) ;
#7698=DIRECTION ( 'NONE',  ( -0.000000000000000000, 1.000000000000000000, -0.000000000000000000 ) ) ;
#7699=ADVANCED_FACE ( 'NONE', ( #28680 ), #12905, .F. ) ;
#7702=DIRECTION ( 'NONE',  ( 0.000000000000000000, 0.000000000000000000, 1.000000000000000000 ) ) ;
#7703=DIRECTION ( 'NONE',  ( -0.000000000000000000, 1.000000000000000000, -0.000000000000000000 ) ) ;
#7705=ORIENTED_EDGE ( 'NONE', *, *, #25271, .F. ) ;
#7749=VERTEX_POINT ( 'NONE', #731 ) ;
#7759=AXIS2_PLACEMENT_3D ( 'NONE', #25766, #32479, #5191 ) ;
#7762=DIRECTION ( 'NONE',  ( 0.000000000000000000, 0.000000000000000000, 1.000000000000000000 ) ) ;
#7770=CARTESIAN_POINT ( 'NONE',  ( 571.1634899080285095, 259.9999999999999432, -199.9999999999981526 ) ) ;
#7771=PLANE ( 'NONE',  #45215 ) ;
#7775=CIRCLE ( 'NONE', #1129, 2.749999999999891642 ) ;
#7791=EDGE_CURVE ( 'NONE', #32511, #21321, #32136, .T. ) ;
#7799=AXIS2_PLACEMENT_3D ( 'NONE', #14200, #4707, #7285 ) ;
#7828=DIRECTION ( 'NONE',  ( -1.000000000000000000, 0.000000000000000000, 0.000000000000000000 ) ) ;
#7835=CARTESIAN_POINT ( 'NONE',  ( 311.1634899080286232, 260.0000000000000000, -199.9999999999963336 ) ) ;
#7864=AXIS2_PLACEMENT_3D ( 'NONE', #4600, #1364, #4829 ) ;
#7904=AXIS2_PLACEMENT_3D ( 'NONE', #6153, #34568, #20917 ) ;
#7908=( LENGTH_UNIT ( ) NAMED_UNIT ( * ) SI_UNIT ( .MILLI., .METRE. ) );
#7928=DIRECTION ( 'NONE',  ( 1.892425610156518354E-16, 1.000000000000000000, -0.000000000000000000 ) ) ;
#7946=DIRECTION ( 'NONE',  ( 0.000000000000000000, 0.000000000000000000, 1.000000000000000000 ) ) ;
#7962=VECTOR ( 'NONE', #5328, 1000.000000000000000 ) ;
#7990=VERTEX_POINT ( 'NONE', #12034 ) ;
#8000=ORIENTED_EDGE ( 'NONE', *, *, #13409, .T. ) ;
#8002=DIRECTION ( 'NONE',  ( -0.000000000000000000, 1.000000000000000000, -0.000000000000000000 ) ) ;
#8006=DIRECTION ( 'NONE',  ( -1.000000000000000000, 0.000000000000000000, 0.000000000000000000 ) ) ;
#8019=CARTESIAN_POINT ( 'NONE',  ( -78.83651009197140525, 260.0000000000000568, -197.2499999999937756 ) ) ;
#8024=AXIS2_PLACEMENT_3D ( 'NONE', #38580, #39271, #35106 ) ;
#8042=VERTEX_POINT ( 'NONE', #33945 ) ;
#8063=EDGE_CURVE ( 'NONE', #17707, #2736, #38007, .T. ) ;
#8069=ORIENTED_EDGE ( 'NONE', *, *, #17979, .F. ) ;
#8072=LINE ( 'NONE', #22134, #38911 ) ;
#8094=EDGE_CURVE ( 'NONE', #27562, #41260, #4087, .T. ) ;
#8110=CARTESIAN_POINT ( 'NONE',  ( -78.83651009197140525, 260.0000000000000568, -193.8809999999935769 ) ) ;
#8113=FACE_OUTER_BOUND ( 'NONE', #9283, .T. ) ;
#8148=LINE ( 'NONE', #35611, #28622 ) ;
#8149=VERTEX_POINT ( 'NONE', #41345 ) ;
#8158=EDGE_LOOP ( 'NONE', ( #11451, #39576, #33005, #25466 ) ) ;
#8217=DIRECTION ( 'NONE',  ( -0.000000000000000000, 1.000000000000000000, -0.000000000000000000 ) ) ;
#8232=LINE ( 'NONE', #25988, #31317 ) ;
#8247=VERTEX_POINT ( 'NONE', #20543 ) ;
#8267=DIRECTION ( 'NONE',  ( 1.892425610156518354E-16, 1.000000000000000000, -0.000000000000000000 ) ) ;
#8273=CARTESIAN_POINT ( 'NONE',  ( -208.8365100919714052, 260.0000000000001137, -199.9999999999926956 ) ) ;
#8288=ORIENTED_EDGE ( 'NONE', *, *, #43103, .T. ) ;
#8294=ORIENTED_EDGE ( 'NONE', *, *, #21009, .T. ) ;
#8297=DIRECTION ( 'NONE',  ( -0.000000000000000000, 1.000000000000000000, -0.000000000000000000 ) ) ;
#8315=ORIENTED_EDGE ( 'NONE', *, *, #4666, .T. ) ;
#8334=CARTESIAN_POINT ( 'NONE',  ( -728.8365100919714905, 256.5000000000001705, -193.8809999999890863 ) ) ;
#8359=AXIS2_PLACEMENT_3D ( 'NONE', #27637, #24392, #13562 ) ;
#8392=LINE ( 'NONE', #32654, #32058 ) ;
#8402=ORIENTED_EDGE ( 'NONE', *, *, #9997, .T. ) ;
#8433=CYLINDRICAL_SURFACE ( 'NONE', #15915, 2.749999999999863665 ) ;
#8435=EDGE_LOOP ( 'NONE', ( #7509, #5329, #24034, #10191 ) ) ;
#8437=CARTESIAN_POINT ( 'NONE',  ( 181.1634899080285948, 256.5000000000000000, -199.9999999999953957 ) ) ;
#8445=DIRECTION ( 'NONE',  ( -0.000000000000000000, 1.000000000000000000, -0.000000000000000000 ) ) ;
#8446=FACE_BOUND ( 'NONE', #28078, .T. ) ;
#8449=AXIS2_PLACEMENT_3D ( 'NONE', #31791, #18190, #14725 ) ;
#8466=LINE ( 'NONE', #12603, #26916 ) ;
#8485=EDGE_LOOP ( 'NONE', ( #43181, #42102 ) ) ;
#8498=CIRCLE ( 'NONE', #26184, 6.118999999999985562 ) ;
#8501=AXIS2_PLACEMENT_3D ( 'NONE', #29131, #4431, #42984 ) ;
#8519=EDGE_LOOP ( 'NONE', ( #8649, #23157, #36994, #27053 ) ) ;
#8544=ADVANCED_FACE ( 'NONE', ( #26017 ), #2452, .F. ) ;
#8552=ORIENTED_EDGE ( 'NONE', *, *, #13735, .F. ) ;
#8577=DIRECTION ( 'NONE',  ( -1.000000000000000000, 0.000000000000000000, 0.000000000000000000 ) ) ;
#8578=CARTESIAN_POINT ( 'NONE',  ( 181.1634899080285948, 256.5000000000000000, -199.9999999999953957 ) ) ;
#8598=EDGE_LOOP ( 'NONE', ( #42155, #35681, #19053, #21427 ) ) ;
#8603=AXIS2_PLACEMENT_3D ( 'NONE', #22949, #33821, #30575 ) ;
#8615=CYLINDRICAL_SURFACE ( 'NONE', #43985, 6.118999999999985562 ) ;
#8616=DIRECTION ( 'NONE',  ( -0.000000000000000000, 1.000000000000000000, -0.000000000000000000 ) ) ;
#8622=EDGE_CURVE ( 'NONE', #30100, #16583, #5920, .T. ) ;
#8637=CIRCLE ( 'NONE', #38879, 8.025000000000003908 ) ;
#8641=CONICAL_SURFACE ( 'NONE', #19593, 8.025000000000003908, 0.7853981633974482790 ) ;
#8647=CARTESIAN_POINT ( 'NONE',  ( -728.8365100919714905, 260.0000000000001705, -199.9999999999890861 ) ) ;
#8649=ORIENTED_EDGE ( 'NONE', *, *, #6020, .F. ) ;
#8712=CONICAL_SURFACE ( 'NONE', #18316, 8.025000000000003908, 0.7853981633974482790 ) ;
#8733=FACE_OUTER_BOUND ( 'NONE', #10414, .T. ) ;
#8740=VERTEX_POINT ( 'NONE', #16554 ) ;
#8791=DIRECTION ( 'NONE',  ( -0.000000000000000000, 1.000000000000000000, -0.000000000000000000 ) ) ;
#8807=DIRECTION ( 'NONE',  ( 0.000000000000000000, 0.000000000000000000, 1.000000000000000000 ) ) ;
#8819=EDGE_LOOP ( 'NONE', ( #15795, #438, #15741, #30393 ) ) ;
#8828=CONICAL_SURFACE ( 'NONE', #13252, 8.025000000000003908, 0.7853981633974410625 ) ;
#8832=DIRECTION ( 'NONE',  ( 1.892425610156518354E-16, 1.000000000000000000, -0.000000000000000000 ) ) ;
#8853=DIRECTION ( 'NONE',  ( -0.000000000000000000, 1.000000000000000000, -0.000000000000000000 ) ) ;
#8857=FACE_OUTER_BOUND ( 'NONE', #25285, .T. ) ;
#8868=ORIENTED_EDGE ( 'NONE', *, *, #12822, .F. ) ;
#8874=EDGE_LOOP ( 'NONE', ( #8288, #10398, #44837, #35620 ) ) ;
#8880=DIRECTION ( 'NONE',  ( 0.000000000000000000, 0.000000000000000000, 1.000000000000000000 ) ) ;
#8882=EDGE_LOOP ( 'NONE', ( #2728, #11684, #41023, #35664 ) ) ;
#8891=CARTESIAN_POINT ( 'NONE',  ( -78.83651009197140525, 260.0000000000000568, -199.9999999999936051 ) ) ;
#8943=ADVANCED_FACE ( 'NONE', ( #3617 ), #27863, .F. ) ;
#8985=AXIS2_PLACEMENT_3D ( 'NONE', #30769, #6274, #23587 ) ;
#9010=CARTESIAN_POINT ( 'NONE',  ( 701.1634899080286232, 256.4999999999999432, -199.9999999999990337 ) ) ;
#9011=DIRECTION ( 'NONE',  ( 0.000000000000000000, 0.7071067811865474617, 0.7071067811865474617 ) ) ;
#9027=FACE_OUTER_BOUND ( 'NONE', #5128, .T. ) ;
#9045=CARTESIAN_POINT ( 'NONE',  ( 187.2824899080286229, 256.5000000000000000, -199.9999999999953957 ) ) ;
#9058=CARTESIAN_POINT ( 'NONE',  ( -598.8365100919716042, 258.0940000000001646, -206.1189999999899385 ) ) ;
#9069=CIRCLE ( 'NONE', #23793, 6.118999999999985562 ) ;
#9082=DIRECTION ( 'NONE',  ( -0.000000000000000000, 1.000000000000000000, -0.000000000000000000 ) ) ;
#9089=EDGE_LOOP ( 'NONE', ( #44420, #44433 ) ) ;
#9095=DIRECTION ( 'NONE',  ( 0.000000000000000000, -1.000000000000000000, 0.000000000000000000 ) ) ;
#9098=DIRECTION ( 'NONE',  ( -0.000000000000000000, 1.000000000000000000, -0.000000000000000000 ) ) ;
#9099=VERTEX_POINT ( 'NONE', #24373 ) ;
#9105=AXIS2_PLACEMENT_3D ( 'NONE', #37162, #1387, #30013 ) ;
#9146=EDGE_CURVE ( 'NONE', #3205, #27542, #3138, .T. ) ;
#9197=EDGE_CURVE ( 'NONE', #42559, #16836, #6309, .T. ) ;
#9199=DIRECTION ( 'NONE',  ( 0.000000000000000000, 0.000000000000000000, 1.000000000000000000 ) ) ;
#9224=ORIENTED_EDGE ( 'NONE', *, *, #19948, .F. ) ;
#9227=CARTESIAN_POINT ( 'NONE',  ( 181.1634899080285948, 256.5000000000000000, -199.9999999999953957 ) ) ;
#9229=FACE_OUTER_BOUND ( 'NONE', #21653, .T. ) ;
#9234=ORIENTED_EDGE ( 'NONE', *, *, #29650, .T. ) ;
#9248=CIRCLE ( 'NONE', #15163, 2.749999999999891642 ) ;
#9258=CIRCLE ( 'NONE', #1143, 8.024999999999948841 ) ;
#9272=VERTEX_POINT ( 'NONE', #43083 ) ;
#9283=EDGE_LOOP ( 'NONE', ( #701, #22471, #1074, #6170 ) ) ;
#9288=DIRECTION ( 'NONE',  ( -0.000000000000000000, 1.000000000000000000, -0.000000000000000000 ) ) ;
#9289=DIRECTION ( 'NONE',  ( 0.000000000000000000, 0.000000000000000000, 1.000000000000000000 ) ) ;
#9306=DIRECTION ( 'NONE',  ( 0.000000000000000000, 0.7071067811865513475, 0.7071067811865435759 ) ) ;
#9313=FACE_OUTER_BOUND ( 'NONE', #15449, .T. ) ;
#9316=CIRCLE ( 'NONE', #1174, 6.118999999999985562 ) ;
#9322=DIRECTION ( 'NONE',  ( -0.000000000000000000, 1.000000000000000000, -0.000000000000000000 ) ) ;
#9342=CARTESIAN_POINT ( 'NONE',  ( -728.8365100919714905, 260.0000000000001705, -199.9999999999890861 ) ) ;
#9343=ORIENTED_EDGE ( 'NONE', *, *, #13311, .F. ) ;
#9359=DIRECTION ( 'NONE',  ( -1.000000000000000000, 0.000000000000000000, 0.000000000000000000 ) ) ;
#9403=DIRECTION ( 'NONE',  ( 0.000000000000000000, 0.000000000000000000, 1.000000000000000000 ) ) ;
#9430=ADVANCED_FACE ( 'NONE', ( #42394 ), #21387, .F. ) ;
#9440=EDGE_CURVE ( 'NONE', #39281, #6808, #18838, .T. ) ;
#9468=ADVANCED_FACE ( 'NONE', ( #42854, #39404 ), #42639, .F. ) ;
#9484=EDGE_CURVE ( 'NONE', #38048, #22371, #599, .T. ) ;
#9514=CARTESIAN_POINT ( 'NONE',  ( -78.83651009197140525, 258.0940000000000509, -199.9999999999936051 ) ) ;
#9530=DIRECTION ( 'NONE',  ( -0.000000000000000000, 1.000000000000000000, -0.000000000000000000 ) ) ;
#9534=DIRECTION ( 'NONE',  ( 0.000000000000000000, 0.000000000000000000, 1.000000000000000000 ) ) ;
#9544=ORIENTED_EDGE ( 'NONE', *, *, #28972, .F. ) ;
#9561=ORIENTED_EDGE ( 'NONE', *, *, #7550, .T. ) ;
#9566=CARTESIAN_POINT ( 'NONE',  ( 701.1634899080286232, 259.9999999999999432, -202.7499999999988916 ) ) ;
#9568=DIRECTION ( 'NONE',  ( -1.000000000000000000, 0.000000000000000000, 0.000000000000000000 ) ) ;
#9572=DIRECTION ( 'NONE',  ( 0.000000000000000000, 0.000000000000000000, 1.000000000000000000 ) ) ;
#9576=CYLINDRICAL_SURFACE ( 'NONE', #20916, 2.749999999999863665 ) ;
#9588=CYLINDRICAL_SURFACE ( 'NONE', #27665, 6.118999999999985562 ) ;
#9606=PLANE ( 'NONE',  #39375 ) ;
#9616=EDGE_LOOP ( 'NONE', ( #32288, #12871 ) ) ;
#9679=EDGE_CURVE ( 'NONE', #26697, #9876, #40318, .T. ) ;
#9682=ORIENTED_EDGE ( 'NONE', *, *, #30903, .F. ) ;
#9734=ADVANCED_FACE ( 'NONE', ( #40740 ), #28470, .F. ) ;
#9737=EDGE_LOOP ( 'NONE', ( #28668, #31558 ) ) ;
#9750=EDGE_CURVE ( 'NONE', #18427, #12174, #22503, .T. ) ;
#9773=ORIENTED_EDGE ( 'NONE', *, *, #5829, .F. ) ;
#9794=CARTESIAN_POINT ( 'NONE',  ( 701.1634899080286232, 259.9999999999999432, -199.9999999999990337 ) ) ;
#9798=DIRECTION ( 'NONE',  ( 0.000000000000000000, 0.7071067811865578978, 0.7071067811865372477 ) ) ;
#9802=AXIS2_PLACEMENT_3D ( 'NONE', #40544, #19503, #33600 ) ;
#9814=FACE_OUTER_BOUND ( 'NONE', #14920, .T. ) ;
#9876=VERTEX_POINT ( 'NONE', #1936 ) ;
#9885=DIRECTION ( 'NONE',  ( 0.000000000000000000, 0.000000000000000000, 1.000000000000000000 ) ) ;
#9887=VERTEX_POINT ( 'NONE', #16039 ) ;
#9924=CARTESIAN_POINT ( 'NONE',  ( -728.8365100919714905, 258.0940000000001646, -199.9999999999890861 ) ) ;
#9935=AXIS2_PLACEMENT_3D ( 'NONE', #40932, #30296, #23125 ) ;
#9945=CARTESIAN_POINT ( 'NONE',  ( 831.1634899080286232, 259.9999999999998863, -199.9999999999999432 ) ) ;
#9946=EDGE_LOOP ( 'NONE', ( #14261, #4783 ) ) ;
#9958=EDGE_LOOP ( 'NONE', ( #15985, #30559, #20793, #31910 ) ) ;
#9961=AXIS2_PLACEMENT_3D ( 'NONE', #24625, #6742, #3052 ) ;
#9970=AXIS2_PLACEMENT_3D ( 'NONE', #44115, #44342, #12698 ) ;
#9997=EDGE_CURVE ( 'NONE', #40519, #32688, #23852, .T. ) ;
#10021=CYLINDRICAL_SURFACE ( 'NONE', #5608, 6.118999999999985562 ) ;
#10028=ADVANCED_FACE ( 'NONE', ( #6323 ), #10021, .F. ) ;
#10080=AXIS2_PLACEMENT_3D ( 'NONE', #9342, #12572, #12358 ) ;
#10088=CARTESIAN_POINT ( 'NONE',  ( -879.9999999999992042, 260.0000000000002274, -179.9999999999999716 ) ) ;
#10093=CARTESIAN_POINT ( 'NONE',  ( -858.8365100919713768, 260.0000000000002274, -199.9999999999881481 ) ) ;
#10105=ORIENTED_EDGE ( 'NONE', *, *, #9679, .F. ) ;
#10116=CARTESIAN_POINT ( 'NONE',  ( 571.1634899080285095, 256.4999999999999432, -199.9999999999981526 ) ) ;
#10119=VERTEX_POINT ( 'NONE', #27800 ) ;
#10124=EDGE_LOOP ( 'NONE', ( #22556, #17858, #39759, #19047 ) ) ;
#10139=LINE ( 'NONE', #38539, #466 ) ;
#10191=ORIENTED_EDGE ( 'NONE', *, *, #3007, .T. ) ;
#10203=DIRECTION ( 'NONE',  ( -1.000000000000000000, 0.000000000000000000, 0.000000000000000000 ) ) ;
#10241=FACE_OUTER_BOUND ( 'NONE', #41389, .T. ) ;
#10292=ORIENTED_EDGE ( 'NONE', *, *, #16475, .T. ) ;
#10324=FACE_OUTER_BOUND ( 'NONE', #34544, .T. ) ;
#10336=DIRECTION ( 'NONE',  ( 0.000000000000000000, 0.000000000000000000, 1.000000000000000000 ) ) ;
#10342=DIRECTION ( 'NONE',  ( 0.000000000000000000, 0.000000000000000000, 1.000000000000000000 ) ) ;
#10357=EDGE_LOOP ( 'NONE', ( #42044, #27787, #16948, #8868 ) ) ;
#10361=DIRECTION ( 'NONE',  ( -0.000000000000000000, 1.000000000000000000, -0.000000000000000000 ) ) ;
#10398=ORIENTED_EDGE ( 'NONE', *, *, #10616, .F. ) ;
#10407=ORIENTED_EDGE ( 'NONE', *, *, #20111, .F. ) ;
#10414=EDGE_LOOP ( 'NONE', ( #3992, #31864, #20259, #413 ) ) ;
#10442=DIRECTION ( 'NONE',  ( 0.000000000000000000, 0.000000000000000000, 1.000000000000000000 ) ) ;
#10481=DIRECTION ( 'NONE',  ( -0.000000000000000000, 1.000000000000000000, -0.000000000000000000 ) ) ;
#10491=DIRECTION ( 'NONE',  ( -0.000000000000000000, 1.000000000000000000, -0.000000000000000000 ) ) ;
#10506=ORIENTED_EDGE ( 'NONE', *, *, #7494, .T. ) ;
#10512=EDGE_CURVE ( 'NONE', #40012, #29996, #12978, .T. ) ;
#10521=DIRECTION ( 'NONE',  ( -0.000000000000000000, 1.000000000000000000, -0.000000000000000000 ) ) ;
#10540=FACE_OUTER_BOUND ( 'NONE', #7526, .T. ) ;
#10545=DIRECTION ( 'NONE',  ( -0.000000000000000000, 1.000000000000000000, -0.000000000000000000 ) ) ;
#10586=VERTEX_POINT ( 'NONE', #39124 ) ;
#10590=EDGE_CURVE ( 'NONE', #13375, #4510, #7475, .T. ) ;
#10592=LINE ( 'NONE', #21445, #30012 ) ;
#10593=DIRECTION ( 'NONE',  ( 0.000000000000000000, -0.000000000000000000, -1.000000000000000000 ) ) ;
#10600=AXIS2_PLACEMENT_3D ( 'NONE', #22623, #44100, #12464 ) ;
#10606=DIRECTION ( 'NONE',  ( 0.000000000000000000, 0.000000000000000000, 1.000000000000000000 ) ) ;
#10607=EDGE_CURVE ( 'NONE', #9887, #27562, #28723, .T. ) ;
#10616=EDGE_CURVE ( 'NONE', #5298, #14461, #32639, .T. ) ;
#10640=VECTOR ( 'NONE', #23044, 999.9999999999998863 ) ;
#10641=CARTESIAN_POINT ( 'NONE',  ( -468.8365100919714337, 256.5000000000001705, -199.9999999999908766 ) ) ;
#10647=ORIENTED_EDGE ( 'NONE', *, *, #12591, .F. ) ;
#10668=CARTESIAN_POINT ( 'NONE',  ( 51.16348990802859475, 260.0000000000000568, -199.9999999999945146 ) ) ;
#10687=ORIENTED_EDGE ( 'NONE', *, *, #40248, .F. ) ;
#10694=VERTEX_POINT ( 'NONE', #15086 ) ;
#10703=CARTESIAN_POINT ( 'NONE',  ( 701.1634899080286232, 258.0939999999999372, -206.1189999999990334 ) ) ;
#10712=LINE ( 'NONE', #38912, #34197 ) ;
#10737=CARTESIAN_POINT ( 'NONE',  ( -468.8365100919714337, 258.0940000000001646, -206.1189999999908764 ) ) ;
#10740=VERTEX_POINT ( 'NONE', #22225 ) ;
#10754=CIRCLE ( 'NONE', #11553, 2.749999999999919176 ) ;
#10778=DIRECTION ( 'NONE',  ( 0.000000000000000000, -0.000000000000000000, -1.000000000000000000 ) ) ;
#10791=ADVANCED_FACE ( 'NONE', ( #5582 ), #8615, .F. ) ;
#10792=VECTOR ( 'NONE', #35067, 1000.000000000000000 ) ;
#10815=VERTEX_POINT ( 'NONE', #43476 ) ;
#10834=EDGE_CURVE ( 'NONE', #11865, #10866, #33673, .T. ) ;
#10849=CARTESIAN_POINT ( 'NONE',  ( 181.1634899080285948, 240.0000000000000284, -199.9999999999953957 ) ) ;
#10866=VERTEX_POINT ( 'NONE', #44152 ) ;
#10881=VERTEX_POINT ( 'NONE', #12735 ) ;
#10882=AXIS2_PLACEMENT_3D ( 'NONE', #37780, #21140, #20219 ) ;
#10912=FACE_BOUND ( 'NONE', #38183, .T. ) ;
#10919=VECTOR ( 'NONE', #23561, 1000.000000000000000 ) ;
#10922=ORIENTED_EDGE ( 'NONE', *, *, #34797, .T. ) ;
#10929=DIRECTION ( 'NONE',  ( -0.000000000000000000, 1.000000000000000000, -0.000000000000000000 ) ) ;
#10936=ORIENTED_EDGE ( 'NONE', *, *, #20487, .T. ) ;
#10949=DIRECTION ( 'NONE',  ( -0.000000000000000000, 1.000000000000000000, -0.000000000000000000 ) ) ;
#10956=DIRECTION ( 'NONE',  ( -0.000000000000000000, 1.000000000000000000, -0.000000000000000000 ) ) ;
#10958=ADVANCED_FACE ( 'NONE', ( #19439, #12518 ), #26592, .F. ) ;
#10995=EDGE_LOOP ( 'NONE', ( #5619, #39126, #23938, #32115 ) ) ;
#11007=DIRECTION ( 'NONE',  ( -1.000000000000000000, 0.000000000000000000, 0.000000000000000000 ) ) ;
#11032=VERTEX_POINT ( 'NONE', #30514 ) ;
#11061=CARTESIAN_POINT ( 'NONE',  ( -468.8365100919714337, 256.5000000000001705, -197.2499999999909619 ) ) ;
#11084=ORIENTED_EDGE ( 'NONE', *, *, #31441, .F. ) ;
#11105=CARTESIAN_POINT ( 'NONE',  ( -728.8365100919714905, 258.0940000000001646, -206.1189999999890574 ) ) ;
#11138=EDGE_LOOP ( 'NONE', ( #25224, #19000 ) ) ;
#11146=EDGE_LOOP ( 'NONE', ( #30743, #44882, #5913, #30986 ) ) ;
#11162=CARTESIAN_POINT ( 'NONE',  ( 831.1634899080286232, 259.9999999999998863, -193.8809999999999718 ) ) ;
#11181=DIRECTION ( 'NONE',  ( 0.000000000000000000, 0.000000000000000000, 1.000000000000000000 ) ) ;
#11187=LINE ( 'NONE', #42362, #11413 ) ;
#11192=DIRECTION ( 'NONE',  ( -1.880165489482579047E-16, -1.000000000000000000, 0.000000000000000000 ) ) ;
#11200=UNCERTAINTY_MEASURE_WITH_UNIT (LENGTH_MEASURE( 1.000000000000000082E-05 ), #7908, 'distance_accuracy_value', 'NONE');
#11221=DIRECTION ( 'NONE',  ( -0.000000000000000000, 1.000000000000000000, -0.000000000000000000 ) ) ;
#11253=EDGE_LOOP ( 'NONE', ( #42446, #22998 ) ) ;
#11284=LINE ( 'NONE', #3679, #4629 ) ;
#11287=ORIENTED_EDGE ( 'NONE', *, *, #34190, .T. ) ;
#11302=CARTESIAN_POINT ( 'NONE',  ( -78.83651009197140525, 240.0000000000000568, -202.7499999999934346 ) ) ;
#11319=ORIENTED_EDGE ( 'NONE', *, *, #9197, .F. ) ;
#11331=DIRECTION ( 'NONE',  ( 0.000000000000000000, 0.000000000000000000, 1.000000000000000000 ) ) ;
#11378=EDGE_CURVE ( 'NONE', #17860, #2952, #5654, .T. ) ;
#11388=CARTESIAN_POINT ( 'NONE',  ( -468.8365100919714337, 260.0000000000001705, -199.9999999999908766 ) ) ;
#11413=VECTOR ( 'NONE', #24810, 1000.000000000000000 ) ;
#11423=CLOSED_SHELL ( 'NONE', ( #6698, #36248, #20743, #36281, #34905, #27494, #43570, #9430, #15719, #9734, #10028, #3510, #44780, #457, #35494, #38156, #36856, #32036, #12495, #8943, #8544, #29549, #24076, #25232, #39746, #41925, #26692, #32290, #10791, #3858, #11998, #2695, #39368, #18093, #32108, #35370, #29138, #13392, #40304, #41964, #5431, #5761, #25253, #13139, #22387, #25015, #43003, #622, #39984, #5757, #35720, #41395, #4947, #30690, #31450, #24426, #44186, #20762, #18479, #22604, #24121, #28696, #26310, #38857, #11985, #746, #38787, #30113, #26143, #9468, #41041, #22772, #1338, #21364, #18251, #18816, #32321, #24106, #40782, #675, #44157, #10958, #30266, #38734, #19870, #40220, #970, #26097, #24052, #42532, #12826, #34846, #20643, #16806, #18789, #19029, #4670, #41534, #20975, #7699, #27691, #33164, #35703, #12565 ) ) ;
#11430=ORIENTED_EDGE ( 'NONE', *, *, #36217, .F. ) ;
#11449=AXIS2_PLACEMENT_3D ( 'NONE', #1730, #5899, #32552 ) ;
#11451=ORIENTED_EDGE ( 'NONE', *, *, #27552, .F. ) ;
#11463=FACE_BOUND ( 'NONE', #26064, .T. ) ;
#11466=VECTOR ( 'NONE', #12373, 1000.000000000000000 ) ;
#11506=AXIS2_PLACEMENT_3D ( 'NONE', #3841, #8217, #28555 ) ;
#11521=DIRECTION ( 'NONE',  ( -0.000000000000000000, 1.000000000000000000, -0.000000000000000000 ) ) ;
#11529=LINE ( 'NONE', #44690, #20457 ) ;
#11537=VECTOR ( 'NONE', #4968, 999.9999999999998863 ) ;
#11553=AXIS2_PLACEMENT_3D ( 'NONE', #10641, #28187, #13262 ) ;
#11568=DIRECTION ( 'NONE',  ( 0.000000000000000000, 0.000000000000000000, 1.000000000000000000 ) ) ;
#11586=CIRCLE ( 'NONE', #44006, 6.118999999999985562 ) ;
#11610=CARTESIAN_POINT ( 'NONE',  ( -208.8365100919714052, 256.5000000000001137, -199.9999999999926956 ) ) ;
#11632=EDGE_CURVE ( 'NONE', #19382, #37578, #26027, .T. ) ;
#11674=ORIENTED_EDGE ( 'NONE', *, *, #22762, .F. ) ;
#11684=ORIENTED_EDGE ( 'NONE', *, *, #18143, .T. ) ;
#11693=CARTESIAN_POINT ( 'NONE',  ( 831.1634899080286232, 259.9999999999998863, -197.2500000000000853 ) ) ;
#11707=CARTESIAN_POINT ( 'NONE',  ( -78.83651009197140525, 260.0000000000000568, -208.0249999999936108 ) ) ;
#11730=ORIENTED_EDGE ( 'NONE', *, *, #40850, .F. ) ;
#11757=DIRECTION ( 'NONE',  ( 0.000000000000000000, 0.000000000000000000, 1.000000000000000000 ) ) ;
#11798=ORIENTED_EDGE ( 'NONE', *, *, #36558, .F. ) ;
#11805=CARTESIAN_POINT ( 'NONE',  ( -208.8365100919714052, 258.0940000000001078, -199.9999999999926956 ) ) ;
#11829=VERTEX_POINT ( 'NONE', #12190 ) ;
#11865=VERTEX_POINT ( 'NONE', #23471 ) ;
#11878=CARTESIAN_POINT ( 'NONE',  ( 571.1634899080285095, 258.0939999999999372, -206.1189999999981239 ) ) ;
#11907=FACE_BOUND ( 'NONE', #15318, .T. ) ;
#11918=CARTESIAN_POINT ( 'NONE',  ( -468.8365100919714337, 260.0000000000001705, -208.0249999999908823 ) ) ;
#11933=CARTESIAN_POINT ( 'NONE',  ( -208.8365100919714052, 240.0000000000000853, -197.2499999999928377 ) ) ;
#11956=CARTESIAN_POINT ( 'NONE',  ( 441.1634899080286232, 256.4999999999999432, -193.8809999999972433 ) ) ;
#11962=CARTESIAN_POINT ( 'NONE',  ( -208.8365100919714052, 260.0000000000001137, -197.2499999999928377 ) ) ;
#11985=ADVANCED_FACE ( 'NONE', ( #13103 ), #26494, .F. ) ;
#11987=AXIS2_PLACEMENT_3D ( 'NONE', #23697, #23475, #20021 ) ;
#11998=ADVANCED_FACE ( 'NONE', ( #42403 ), #8641, .F. ) ;
#12000=ORIENTED_EDGE ( 'NONE', *, *, #18568, .T. ) ;
#12019=VERTEX_POINT ( 'NONE', #14015 ) ;
#12021=CIRCLE ( 'NONE', #15706, 6.118999999999985562 ) ;
#12028=CARTESIAN_POINT ( 'NONE',  ( -468.8365100919714337, 256.5000000000001705, -199.9999999999908766 ) ) ;
#12034=CARTESIAN_POINT ( 'NONE',  ( 51.16348990802859475, 256.5000000000000568, -193.8809999999945148 ) ) ;
#12074=ORIENTED_EDGE ( 'NONE', *, *, #43019, .T. ) ;
#12121=CARTESIAN_POINT ( 'NONE',  ( 57.28248990802860163, 256.5000000000000568, -199.9999999999945146 ) ) ;
#12122=CARTESIAN_POINT ( 'NONE',  ( -728.8365100919714905, 260.0000000000001705, -191.9749999999891372 ) ) ;
#12138=CIRCLE ( 'NONE', #22432, 6.118999999999985562 ) ;
#12172=ORIENTED_EDGE ( 'NONE', *, *, #16501, .T. ) ;
#12174=VERTEX_POINT ( 'NONE', #35014 ) ;
#12181=CIRCLE ( 'NONE', #23955, 6.119000000000013095 ) ;
#12190=CARTESIAN_POINT ( 'NONE',  ( 701.1634899080286232, 256.4999999999999432, -193.8809999999990623 ) ) ;
#12193=DIRECTION ( 'NONE',  ( -0.000000000000000000, 1.000000000000000000, -0.000000000000000000 ) ) ;
#12199=DIRECTION ( 'NONE',  ( 0.000000000000000000, 0.000000000000000000, 1.000000000000000000 ) ) ;
#12240=ORIENTED_EDGE ( 'NONE', *, *, #28933, .T. ) ;
#12242=DIRECTION ( 'NONE',  ( 0.000000000000000000, 0.000000000000000000, 1.000000000000000000 ) ) ;
#12255=FACE_OUTER_BOUND ( 'NONE', #8819, .T. ) ;
#12284=EDGE_LOOP ( 'NONE', ( #39000, #7644, #37494, #10105 ) ) ;
#12287=EDGE_CURVE ( 'NONE', #33219, #32511, #2701, .T. ) ;
#12298=VERTEX_POINT ( 'NONE', #23921 ) ;
#12309=EDGE_LOOP ( 'NONE', ( #26291, #25022, #42835, #19145 ) ) ;
#12318=DIRECTION ( 'NONE',  ( 0.000000000000000000, 0.000000000000000000, 1.000000000000000000 ) ) ;
#12332=CARTESIAN_POINT ( 'NONE',  ( 441.1634899080286232, 256.4999999999999432, -199.9999999999972431 ) ) ;
#12347=VERTEX_POINT ( 'NONE', #28784 ) ;
#12354=DIRECTION ( 'NONE',  ( -0.000000000000000000, 1.000000000000000000, -0.000000000000000000 ) ) ;
#12358=DIRECTION ( 'NONE',  ( 0.000000000000000000, 0.000000000000000000, 1.000000000000000000 ) ) ;
#12373=DIRECTION ( 'NONE',  ( 0.000000000000000000, 0.000000000000000000, 1.000000000000000000 ) ) ;
#12413=FACE_OUTER_BOUND ( 'NONE', #9958, .T. ) ;
#12435=VERTEX_POINT ( 'NONE', #29462 ) ;
#12446=CARTESIAN_POINT ( 'NONE',  ( -462.7175100919714055, 256.5000000000001705, -199.9999999999908766 ) ) ;
#12448=ORIENTED_EDGE ( 'NONE', *, *, #33669, .F. ) ;
#12457=ORIENTED_EDGE ( 'NONE', *, *, #16521, .T. ) ;
#12460=VERTEX_POINT ( 'NONE', #17933 ) ;
#12464=DIRECTION ( 'NONE',  ( 0.000000000000000000, 0.000000000000000000, 1.000000000000000000 ) ) ;
#12495=ADVANCED_FACE ( 'NONE', ( #827 ), #45437, .F. ) ;
#12499=DIRECTION ( 'NONE',  ( -1.000000000000000000, 0.000000000000000000, 0.000000000000000000 ) ) ;
#12512=ORIENTED_EDGE ( 'NONE', *, *, #41538, .T. ) ;
#12518=FACE_OUTER_BOUND ( 'NONE', #11253, .T. ) ;
#12520=DIRECTION ( 'NONE',  ( 1.000000000000000000, -1.892425610156518354E-16, 0.000000000000000000 ) ) ;
#12521=EDGE_LOOP ( 'NONE', ( #9544, #26284 ) ) ;
#12524=CARTESIAN_POINT ( 'NONE',  ( 51.16348990802859475, 258.0940000000000509, -193.8809999999945433 ) ) ;
#12533=EDGE_CURVE ( 'NONE', #37578, #41429, #39577, .T. ) ;
#12544=DIRECTION ( 'NONE',  ( -0.000000000000000000, -0.000000000000000000, -1.000000000000000000 ) ) ;
#12554=ORIENTED_EDGE ( 'NONE', *, *, #5197, .F. ) ;
#12565=ADVANCED_FACE ( 'NONE', ( #43323 ), #37336, .F. ) ;
#12572=DIRECTION ( 'NONE',  ( -0.000000000000000000, 1.000000000000000000, -0.000000000000000000 ) ) ;
#12575=LINE ( 'NONE', #26879, #41120 ) ;
#12591=EDGE_CURVE ( 'NONE', #32411, #45239, #21089, .T. ) ;
#12596=DIRECTION ( 'NONE',  ( 8.659560562354900811E-17, 0.7071067811865501263, -0.7071067811865449082 ) ) ;
#12603=CARTESIAN_POINT ( 'NONE',  ( -208.8365100919714052, 260.0000000000001137, -208.0249999999927013 ) ) ;
#12606=ORIENTED_EDGE ( 'NONE', *, *, #21615, .T. ) ;
#12621=ORIENTED_EDGE ( 'NONE', *, *, #1578, .T. ) ;
#12647=ORIENTED_EDGE ( 'NONE', *, *, #24620, .T. ) ;
#12660=ORIENTED_EDGE ( 'NONE', *, *, #40248, .T. ) ;
#12680=DIRECTION ( 'NONE',  ( -0.000000000000000000, 1.000000000000000000, -0.000000000000000000 ) ) ;
#12685=ORIENTED_EDGE ( 'NONE', *, *, #39938, .F. ) ;
#12698=DIRECTION ( 'NONE',  ( 0.000000000000000000, 0.000000000000000000, 1.000000000000000000 ) ) ;
#12701=DIRECTION ( 'NONE',  ( -0.000000000000000000, 1.000000000000000000, -0.000000000000000000 ) ) ;
#12721=ORIENTED_EDGE ( 'NONE', *, *, #42537, .T. ) ;
#12735=CARTESIAN_POINT ( 'NONE',  ( -78.83651009197140525, 256.5000000000000568, -206.1189999999936049 ) ) ;
#12761=DIRECTION ( 'NONE',  ( -0.000000000000000000, -0.000000000000000000, -1.000000000000000000 ) ) ;
#12797=CARTESIAN_POINT ( 'NONE',  ( -858.8365100919713768, 258.0940000000002215, -199.9999999999881481 ) ) ;
#12822=EDGE_CURVE ( 'NONE', #11865, #27126, #29003, .T. ) ;
#12826=ADVANCED_FACE ( 'NONE', ( #22068 ), #39408, .F. ) ;
#12871=ORIENTED_EDGE ( 'NONE', *, *, #4666, .F. ) ;
#12886=DIRECTION ( 'NONE',  ( 0.000000000000000000, 0.000000000000000000, 1.000000000000000000 ) ) ;
#12890=CIRCLE ( 'NONE', #16593, 8.024999999999948841 ) ;
#12902=AXIS2_PLACEMENT_3D ( 'NONE', #9010, #23080, #26778 ) ;
#12903=ORIENTED_EDGE ( 'NONE', *, *, #15105, .T. ) ;
#12905=CONICAL_SURFACE ( 'NONE', #8501, 8.024999999999948841, 0.7853981633974337351 ) ;
#12912=AXIS2_PLACEMENT_3D ( 'NONE', #13796, #21168, #7320 ) ;
#12917=CIRCLE ( 'NONE', #40230, 6.118999999999985562 ) ;
#12931=LINE ( 'NONE', #2523, #2586 ) ;
#12938=DIRECTION ( 'NONE',  ( -0.000000000000000000, 1.000000000000000000, -0.000000000000000000 ) ) ;
#12957=CONICAL_SURFACE ( 'NONE', #7799, 8.024999999999948841, 0.7853981633974337351 ) ;
#12961=DIRECTION ( 'NONE',  ( -0.000000000000000000, 1.000000000000000000, -0.000000000000000000 ) ) ;
#12962=ORIENTED_EDGE ( 'NONE', *, *, #1239, .F. ) ;
#12965=EDGE_LOOP ( 'NONE', ( #19216, #2436 ) ) ;
#12978=CIRCLE ( 'NONE', #38804, 8.024999999999948841 ) ;
#12982=CYLINDRICAL_SURFACE ( 'NONE', #28553, 2.749999999999863665 ) ;
#12984=CARTESIAN_POINT ( 'NONE',  ( 879.9999999999992042, 259.9999999999998863, -179.9999999999999716 ) ) ;
#12996=CARTESIAN_POINT ( 'NONE',  ( 701.1634899080286232, 259.9999999999999432, -199.9999999999990337 ) ) ;
#13018=ORIENTED_EDGE ( 'NONE', *, *, #18488, .T. ) ;
#13050=VECTOR ( 'NONE', #39474, 1000.000000000000000 ) ;
#13051=CARTESIAN_POINT ( 'NONE',  ( -858.8365100919713768, 240.0000000000002274, -199.9999999999881481 ) ) ;
#13057=VECTOR ( 'NONE', #7196, 1000.000000000000000 ) ;
#13068=DIRECTION ( 'NONE',  ( 0.000000000000000000, 0.000000000000000000, 1.000000000000000000 ) ) ;
#13072=EDGE_CURVE ( 'NONE', #41197, #36773, #9316, .T. ) ;
#13079=EDGE_LOOP ( 'NONE', ( #45225, #12512, #38631, #30076 ) ) ;
#13080=CIRCLE ( 'NONE', #16773, 2.749999999999919176 ) ;
#13089=ORIENTED_EDGE ( 'NONE', *, *, #41855, .F. ) ;
#13103=FACE_OUTER_BOUND ( 'NONE', #32616, .T. ) ;
#13118=CARTESIAN_POINT ( 'NONE',  ( 701.1634899080286232, 259.9999999999999432, -197.2499999999991758 ) ) ;
#13123=CIRCLE ( 'NONE', #43357, 2.749999999999835687 ) ;
#13130=ORIENTED_EDGE ( 'NONE', *, *, #1848, .T. ) ;
#13139=ADVANCED_FACE ( 'NONE', ( #2174 ), #4971, .F. ) ;
#13158=CYLINDRICAL_SURFACE ( 'NONE', #32734, 6.119000000000013095 ) ;
#13200=EDGE_LOOP ( 'NONE', ( #32735, #2429, #33922, #15494 ) ) ;
#13211=EDGE_LOOP ( 'NONE', ( #18034, #33343 ) ) ;
#13240=CARTESIAN_POINT ( 'NONE',  ( 701.1634899080286232, 259.9999999999999432, -206.1189999999990334 ) ) ;
#13250=ORIENTED_EDGE ( 'NONE', *, *, #17953, .F. ) ;
#13252=AXIS2_PLACEMENT_3D ( 'NONE', #1099, #9098, #43586 ) ;
#13262=DIRECTION ( 'NONE',  ( 0.000000000000000000, 0.000000000000000000, 1.000000000000000000 ) ) ;
#13275=DIRECTION ( 'NONE',  ( -0.000000000000000000, 1.000000000000000000, -0.000000000000000000 ) ) ;
#13282=DIRECTION ( 'NONE',  ( -0.000000000000000000, 1.000000000000000000, -0.000000000000000000 ) ) ;
#13295=CARTESIAN_POINT ( 'NONE',  ( 831.1634899080286232, 256.4999999999998863, -199.9999999999999432 ) ) ;
#13311=EDGE_CURVE ( 'NONE', #34024, #22852, #31473, .T. ) ;
#13332=EDGE_LOOP ( 'NONE', ( #7533, #14567, #8402, #35438 ) ) ;
#13344=EDGE_LOOP ( 'NONE', ( #25228, #25600, #12000, #16372 ) ) ;
#13364=ADVANCED_BREP_SHAPE_REPRESENTATION ( '', ( #2718, #26858 ), #32791 ) ;
#13375=VERTEX_POINT ( 'NONE', #40322 ) ;
#13386=AXIS2_PLACEMENT_3D ( 'NONE', #43265, #10956, #22022 ) ;
#13392=ADVANCED_FACE ( 'NONE', ( #5185 ), #19271, .F. ) ;
#13409=EDGE_CURVE ( 'NONE', #22607, #42507, #37280, .T. ) ;
#13421=CYLINDRICAL_SURFACE ( 'NONE', #33810, 6.118999999999985562 ) ;
#13445=EDGE_CURVE ( 'NONE', #41260, #27562, #21154, .T. ) ;
#13448=AXIS2_PLACEMENT_3D ( 'NONE', #6563, #27812, #24331 ) ;
#13457=DIRECTION ( 'NONE',  ( -1.000000000000000000, 1.892425610156518354E-16, 0.000000000000000000 ) ) ;
#13467=EDGE_LOOP ( 'NONE', ( #45009, #19011, #29556, #13089 ) ) ;
#13495=LINE ( 'NONE', #31268, #42324 ) ;
#13499=CARTESIAN_POINT ( 'NONE',  ( -598.8365100919716042, 260.0000000000001705, -206.1189999999899385 ) ) ;
#13505=AXIS2_PLACEMENT_3D ( 'NONE', #37290, #23867, #2184 ) ;
#13531=ORIENTED_EDGE ( 'NONE', *, *, #919, .F. ) ;
#13540=CIRCLE ( 'NONE', #10600, 8.025000000000003908 ) ;
#13562=DIRECTION ( 'NONE',  ( 0.000000000000000000, 0.000000000000000000, 1.000000000000000000 ) ) ;
#13565=DIRECTION ( 'NONE',  ( -1.000000000000000000, 0.000000000000000000, 0.000000000000000000 ) ) ;
#13600=VERTEX_POINT ( 'NONE', #34507 ) ;
#13614=AXIS2_PLACEMENT_3D ( 'NONE', #39947, #682, #21688 ) ;
#13636=ORIENTED_EDGE ( 'NONE', *, *, #109, .T. ) ;
#13647=CONICAL_SURFACE ( 'NONE', #24710, 8.025000000000003908, 0.7853981633974482790 ) ;
#13658=DIRECTION ( 'NONE',  ( 0.000000000000000000, 0.000000000000000000, 1.000000000000000000 ) ) ;
#13678=AXIS2_PLACEMENT_3D ( 'NONE', #36132, #35660, #4276 ) ;
#13710=EDGE_CURVE ( 'NONE', #25447, #15531, #28025, .T. ) ;
#13735=EDGE_CURVE ( 'NONE', #30554, #42559, #37741, .T. ) ;
#13736=CARTESIAN_POINT ( 'NONE',  ( 831.1634899080286232, 259.9999999999998863, -191.9749999999999943 ) ) ;
#13758=DIRECTION ( 'NONE',  ( 0.000000000000000000, -0.000000000000000000, -1.000000000000000000 ) ) ;
#13767=CARTESIAN_POINT ( 'NONE',  ( -858.8365100919713768, 260.0000000000002274, -208.0249999999880970 ) ) ;
#13796=CARTESIAN_POINT ( 'NONE',  ( -598.8365100919716042, 260.0000000000001705, -199.9999999999899671 ) ) ;
#13799=CARTESIAN_POINT ( 'NONE',  ( 441.1634899080286232, 256.4999999999999432, -197.2499999999973284 ) ) ;
#13807=CYLINDRICAL_SURFACE ( 'NONE', #29383, 6.118999999999985562 ) ;
#13827=EDGE_LOOP ( 'NONE', ( #24770, #32740 ) ) ;
#13842=DIRECTION ( 'NONE',  ( -1.000000000000000000, 0.000000000000000000, 0.000000000000000000 ) ) ;
#13843=VECTOR ( 'NONE', #44048, 1000.000000000000000 ) ;
#13916=FACE_BOUND ( 'NONE', #40906, .T. ) ;
#13947=VERTEX_POINT ( 'NONE', #28728 ) ;
#13966=CARTESIAN_POINT ( 'NONE',  ( -78.83651009197140525, 260.0000000000000568, -199.9999999999936051 ) ) ;
#13988=CARTESIAN_POINT ( 'NONE',  ( -858.8365100919713768, 256.5000000000002274, -206.1189999999881479 ) ) ;
#13993=EDGE_CURVE ( 'NONE', #26697, #34351, #38109, .T. ) ;
#14015=CARTESIAN_POINT ( 'NONE',  ( -78.83651009197140525, 258.0940000000000509, -206.1189999999936049 ) ) ;
#14023=EDGE_CURVE ( 'NONE', #18427, #40312, #33680, .T. ) ;
#14040=DIRECTION ( 'NONE',  ( -0.000000000000000000, 1.000000000000000000, -0.000000000000000000 ) ) ;
#14051=CARTESIAN_POINT ( 'NONE',  ( 441.1634899080286232, 259.9999999999999432, -202.7499999999971010 ) ) ;
#14066=DIRECTION ( 'NONE',  ( -1.000000000000000000, 1.892425610156518354E-16, -0.000000000000000000 ) ) ;
#14082=CARTESIAN_POINT ( 'NONE',  ( 441.1634899080286232, 258.0939999999999372, -199.9999999999972431 ) ) ;
#14096=EDGE_LOOP ( 'NONE', ( #41830, #18102, #4002, #35850 ) ) ;
#14116=PLANE ( 'NONE',  #32982 ) ;
#14130=DIRECTION ( 'NONE',  ( -1.000000000000000000, 0.000000000000000000, 0.000000000000000000 ) ) ;
#14162=ORIENTED_EDGE ( 'NONE', *, *, #42537, .F. ) ;
#14173=CARTESIAN_POINT ( 'NONE',  ( -78.83651009197140525, 256.5000000000000568, -199.9999999999936051 ) ) ;
#14194=CARTESIAN_POINT ( 'NONE',  ( -858.8365100919713768, 260.0000000000002274, -191.9749999999881993 ) ) ;
#14197=AXIS2_PLACEMENT_3D ( 'NONE', #10093, #27189, #23925 ) ;
#14200=CARTESIAN_POINT ( 'NONE',  ( -598.8365100919716042, 260.0000000000001705, -199.9999999999899671 ) ) ;
#14252=DIRECTION ( 'NONE',  ( 1.892425610156518354E-16, 1.000000000000000000, -0.000000000000000000 ) ) ;
#14259=CARTESIAN_POINT ( 'NONE',  ( -598.8365100919716042, 260.0000000000001705, -191.9749999999900183 ) ) ;
#14261=ORIENTED_EDGE ( 'NONE', *, *, #12591, .T. ) ;
#14267=ORIENTED_EDGE ( 'NONE', *, *, #14801, .T. ) ;
#14334=EDGE_CURVE ( 'NONE', #17860, #18427, #10592, .T. ) ;
#14345=CARTESIAN_POINT ( 'NONE',  ( -728.8365100919714905, 260.0000000000001705, -199.9999999999890861 ) ) ;
#14356=CARTESIAN_POINT ( 'NONE',  ( 701.1634899080286232, 239.9999999999999147, -202.7499999999988916 ) ) ;
#14364=AXIS2_PLACEMENT_3D ( 'NONE', #996, #28737, #39139 ) ;
#14394=CONICAL_SURFACE ( 'NONE', #1837, 8.025000000000003908, 0.7853981633974428389 ) ;
#14399=AXIS2_PLACEMENT_3D ( 'NONE', #14082, #42029, #28258 ) ;
#14400=VERTEX_POINT ( 'NONE', #31381 ) ;
#14419=CARTESIAN_POINT ( 'NONE',  ( 571.1634899080285095, 259.9999999999999432, -208.0249999999981014 ) ) ;
#14438=VECTOR ( 'NONE', #10521, 1000.000000000000000 ) ;
#14451=AXIS2_PLACEMENT_3D ( 'NONE', #8647, #19466, #19036 ) ;
#14457=AXIS2_PLACEMENT_3D ( 'NONE', #12121, #9095, #26203 ) ;
#14461=VERTEX_POINT ( 'NONE', #42236 ) ;
#14468=VERTEX_POINT ( 'NONE', #3443 ) ;
#14473=AXIS2_PLACEMENT_3D ( 'NONE', #1486, #22736, #19728 ) ;
#14474=CARTESIAN_POINT ( 'NONE',  ( 571.1634899080285095, 239.9999999999999432, -199.9999999999981526 ) ) ;
#14477=DIRECTION ( 'NONE',  ( 0.000000000000000000, 0.000000000000000000, 1.000000000000000000 ) ) ;
#14481=LINE ( 'NONE', #6843, #36346 ) ;
#14493=VECTOR ( 'NONE', #21717, 1000.000000000000000 ) ;
#14511=VECTOR ( 'NONE', #32420, 1000.000000000000000 ) ;
#14520=EDGE_CURVE ( 'NONE', #17994, #29032, #6426, .T. ) ;
#14536=DIRECTION ( 'NONE',  ( 1.892425610156518354E-16, 1.000000000000000000, -0.000000000000000000 ) ) ;
#14561=AXIS2_PLACEMENT_3D ( 'NONE', #22071, #25074, #28554 ) ;
#14567=ORIENTED_EDGE ( 'NONE', *, *, #4052, .F. ) ;
#14587=AXIS2_PLACEMENT_3D ( 'NONE', #25052, #44415, #33800 ) ;
#14592=DIRECTION ( 'NONE',  ( 0.000000000000000000, -1.000000000000000000, 0.000000000000000000 ) ) ;
#14647=DIRECTION ( 'NONE',  ( -0.000000000000000000, 1.000000000000000000, -0.000000000000000000 ) ) ;
#14682=DIRECTION ( 'NONE',  ( -1.000000000000000000, 0.000000000000000000, 0.000000000000000000 ) ) ;
#14699=CARTESIAN_POINT ( 'NONE',  ( 441.1634899080286232, 256.4999999999999432, -199.9999999999972431 ) ) ;
#14707=DIRECTION ( 'NONE',  ( 1.892425610156518354E-16, 1.000000000000000000, -0.000000000000000000 ) ) ;
#14712=DIRECTION ( 'NONE',  ( -0.000000000000000000, 1.000000000000000000, -0.000000000000000000 ) ) ;
#14725=DIRECTION ( 'NONE',  ( 0.000000000000000000, 0.000000000000000000, 1.000000000000000000 ) ) ;
#14765=FACE_OUTER_BOUND ( 'NONE', #36865, .T. ) ;
#14771=EDGE_CURVE ( 'NONE', #5387, #18328, #8637, .T. ) ;
#14801=EDGE_CURVE ( 'NONE', #30680, #29342, #21912, .T. ) ;
#14834=LINE ( 'NONE', #26105, #5100 ) ;
#14852=CARTESIAN_POINT ( 'NONE',  ( 701.1634899080286232, 259.9999999999999432, -199.9999999999990337 ) ) ;
#14904=VERTEX_POINT ( 'NONE', #663 ) ;
#14911=CIRCLE ( 'NONE', #8985, 8.024999999999948841 ) ;
#14920=EDGE_LOOP ( 'NONE', ( #43306, #20670, #32029, #19435 ) ) ;
#14926=CARTESIAN_POINT ( 'NONE',  ( -468.8365100919714337, 256.5000000000001705, -199.9999999999908766 ) ) ;
#14931=FACE_BOUND ( 'NONE', #44148, .T. ) ;
#14940=LINE ( 'NONE', #8019, #45167 ) ;
#14947=DIRECTION ( 'NONE',  ( -0.000000000000000000, 1.000000000000000000, -0.000000000000000000 ) ) ;
#14983=FACE_OUTER_BOUND ( 'NONE', #39848, .T. ) ;
#14986=ORIENTED_EDGE ( 'NONE', *, *, #26602, .T. ) ;
#15023=CIRCLE ( 'NONE', #38625, 6.118999999999985562 ) ;
#15027=DIRECTION ( 'NONE',  ( -0.000000000000000000, 1.000000000000000000, -0.000000000000000000 ) ) ;
#15029=DIRECTION ( 'NONE',  ( 0.000000000000000000, 0.000000000000000000, 1.000000000000000000 ) ) ;
#15052=PLANE ( 'NONE',  #18088 ) ;
#15055=AXIS2_PLACEMENT_3D ( 'NONE', #43491, #29419, #11181 ) ;
#15086=CARTESIAN_POINT ( 'NONE',  ( -78.83651009197140525, 256.5000000000000568, -197.2499999999937188 ) ) ;
#15105=EDGE_CURVE ( 'NONE', #27542, #4510, #21924, .T. ) ;
#15111=CIRCLE ( 'NONE', #32038, 2.749999999999863665 ) ;
#15117=FACE_OUTER_BOUND ( 'NONE', #24312, .T. ) ;
#15149=ORIENTED_EDGE ( 'NONE', *, *, #40478, .F. ) ;
#15163=AXIS2_PLACEMENT_3D ( 'NONE', #24899, #4573, #18665 ) ;
#15207=AXIS2_PLACEMENT_3D ( 'NONE', #4524, #21844, #4744 ) ;
#15223=AXIS2_PLACEMENT_3D ( 'NONE', #32930, #12354, #43742 ) ;
#15238=CARTESIAN_POINT ( 'NONE',  ( 441.1634899080286232, 259.9999999999999432, -191.9749999999972374 ) ) ;
#15240=ORIENTED_EDGE ( 'NONE', *, *, #43518, .F. ) ;
#15242=AXIS2_PLACEMENT_3D ( 'NONE', #14926, #36162, #373 ) ;
#15318=EDGE_LOOP ( 'NONE', ( #1088, #26857 ) ) ;
#15333=EDGE_CURVE ( 'NONE', #34117, #19382, #21193, .T. ) ;
#15337=DIRECTION ( 'NONE',  ( -0.000000000000000000, 1.000000000000000000, -0.000000000000000000 ) ) ;
#15388=DIRECTION ( 'NONE',  ( -1.000000000000000000, 0.000000000000000000, 0.000000000000000000 ) ) ;
#15389=EDGE_CURVE ( 'NONE', #10881, #12019, #44975, .T. ) ;
#15449=EDGE_LOOP ( 'NONE', ( #32787, #27682, #7146, #23055 ) ) ;
#15468=FACE_OUTER_BOUND ( 'NONE', #38078, .T. ) ;
#15494=ORIENTED_EDGE ( 'NONE', *, *, #7791, .F. ) ;
#15524=LINE ( 'NONE', #22884, #7962 ) ;
#15531=VERTEX_POINT ( 'NONE', #38490 ) ;
#15539=CARTESIAN_POINT ( 'NONE',  ( -208.8365100919714052, 260.0000000000001137, -199.9999999999926956 ) ) ;
#15563=CYLINDRICAL_SURFACE ( 'NONE', #14451, 6.118999999999985562 ) ;
#15580=EDGE_LOOP ( 'NONE', ( #30005, #31715 ) ) ;
#15584=FACE_OUTER_BOUND ( 'NONE', #10124, .T. ) ;
#15586=VERTEX_POINT ( 'NONE', #31328 ) ;
#15656=AXIS2_PLACEMENT_3D ( 'NONE', #4748, #8445, #23640 ) ;
#15658=DIRECTION ( 'NONE',  ( -0.000000000000000000, 1.000000000000000000, -0.000000000000000000 ) ) ;
#15675=CYLINDRICAL_SURFACE ( 'NONE', #7864, 6.118999999999985562 ) ;
#15700=DIRECTION ( 'NONE',  ( 0.000000000000000000, 0.000000000000000000, 1.000000000000000000 ) ) ;
#15706=AXIS2_PLACEMENT_3D ( 'NONE', #3847, #24611, #38728 ) ;
#15719=ADVANCED_FACE ( 'NONE', ( #39658 ), #1288, .F. ) ;
#15741=ORIENTED_EDGE ( 'NONE', *, *, #10512, .T. ) ;
#15761=DIRECTION ( 'NONE',  ( 0.000000000000000000, 0.000000000000000000, 1.000000000000000000 ) ) ;
#15776=DIRECTION ( 'NONE',  ( -1.000000000000000000, 0.000000000000000000, 0.000000000000000000 ) ) ;
#15780=DIRECTION ( 'NONE',  ( 0.000000000000000000, 0.000000000000000000, 1.000000000000000000 ) ) ;
#15781=AXIS2_PLACEMENT_3D ( 'NONE', #4917, #19445, #15761 ) ;
#15795=ORIENTED_EDGE ( 'NONE', *, *, #34190, .F. ) ;
#15820=VECTOR ( 'NONE', #26231, 1000.000000000000000 ) ;
#15831=( GEOMETRIC_REPRESENTATION_CONTEXT ( 3 ) GLOBAL_UNCERTAINTY_ASSIGNED_CONTEXT ( ( #11200 ) ) GLOBAL_UNIT_ASSIGNED_CONTEXT ( ( #7908, #36065, #32827 ) ) REPRESENTATION_CONTEXT ( 'NONE', 'WORKASPACE' ) );
#15840=ORIENTED_EDGE ( 'NONE', *, *, #17010, .F. ) ;
#15852=CIRCLE ( 'NONE', #41683, 8.024999999999948841 ) ;
#15915=AXIS2_PLACEMENT_3D ( 'NONE', #4736, #5633, #30338 ) ;
#15924=ORIENTED_EDGE ( 'NONE', *, *, #16239, .F. ) ;
#15951=AXIS2_PLACEMENT_3D ( 'NONE', #1134, #8297, #39954 ) ;
#15952=CARTESIAN_POINT ( 'NONE',  ( -338.8365100919713200, 260.0000000000001137, -191.9749999999917804 ) ) ;
#15984=EDGE_CURVE ( 'NONE', #9272, #30100, #38501, .T. ) ;
#15985=ORIENTED_EDGE ( 'NONE', *, *, #25000, .F. ) ;
#15998=DIRECTION ( 'NONE',  ( 8.659560562354807133E-17, 0.7071067811865578978, -0.7071067811865372477 ) ) ;
#16006=AXIS2_PLACEMENT_3D ( 'NONE', #21229, #21453, #28152 ) ;
#16039=CARTESIAN_POINT ( 'NONE',  ( 831.1634899080286232, 256.4999999999998863, -193.8809999999999718 ) ) ;
#16065=CARTESIAN_POINT ( 'NONE',  ( 311.1634899080286232, 256.5000000000000000, -199.9999999999963336 ) ) ;
#16080=AXIS2_PLACEMENT_3D ( 'NONE', #11610, #4662, #17850 ) ;
#16088=ORIENTED_EDGE ( 'NONE', *, *, #6335, .F. ) ;
#16101=DIRECTION ( 'NONE',  ( 0.000000000000000000, 0.000000000000000000, 1.000000000000000000 ) ) ;
#16114=CARTESIAN_POINT ( 'NONE',  ( -728.8365100919714905, 260.0000000000001705, -199.9999999999890861 ) ) ;
#16123=EDGE_LOOP ( 'NONE', ( #40980, #1269, #42885, #43298 ) ) ;
#16126=CARTESIAN_POINT ( 'NONE',  ( -858.8365100919713768, 260.0000000000002274, -206.1189999999881479 ) ) ;
#16134=EDGE_LOOP ( 'NONE', ( #32096, #16837, #12621, #19213 ) ) ;
#16149=ORIENTED_EDGE ( 'NONE', *, *, #30641, .T. ) ;
#16151=DIRECTION ( 'NONE',  ( -0.000000000000000000, 1.000000000000000000, -0.000000000000000000 ) ) ;
#16163=DIRECTION ( 'NONE',  ( 0.000000000000000000, 0.000000000000000000, 1.000000000000000000 ) ) ;
#16227=DIRECTION ( 'NONE',  ( 0.000000000000000000, 0.000000000000000000, 1.000000000000000000 ) ) ;
#16234=EDGE_CURVE ( 'NONE', #11032, #9887, #23737, .T. ) ;
#16239=EDGE_CURVE ( 'NONE', #11829, #44849, #3862, .T. ) ;
#16266=DIRECTION ( 'NONE',  ( 8.659560562354932858E-17, 0.7071067811865474617, -0.7071067811865474617 ) ) ;
#16273=DIRECTION ( 'NONE',  ( -0.000000000000000000, 1.000000000000000000, -0.000000000000000000 ) ) ;
#16289=CYLINDRICAL_SURFACE ( 'NONE', #33520, 2.749999999999863665 ) ;
#16295=CARTESIAN_POINT ( 'NONE',  ( -78.83651009197140525, 260.0000000000000568, -191.9749999999935994 ) ) ;
#16342=ORIENTED_EDGE ( 'NONE', *, *, #409, .F. ) ;
#16360=LINE ( 'NONE', #36706, #10640 ) ;
#16362=ORIENTED_EDGE ( 'NONE', *, *, #9750, .T. ) ;
#16367=APPLICATION_CONTEXT ( 'automotive_design' ) ;
#16372=ORIENTED_EDGE ( 'NONE', *, *, #21570, .T. ) ;
#16375=ORIENTED_EDGE ( 'NONE', *, *, #26602, .F. ) ;
#16389=DIRECTION ( 'NONE',  ( 0.000000000000000000, 0.000000000000000000, 1.000000000000000000 ) ) ;
#16415=CARTESIAN_POINT ( 'NONE',  ( 311.1634899080286232, 260.0000000000000000, -202.7499999999961915 ) ) ;
#16419=ORIENTED_EDGE ( 'NONE', *, *, #31104, .F. ) ;
#16437=ORIENTED_EDGE ( 'NONE', *, *, #24177, .T. ) ;
#16443=EDGE_CURVE ( 'NONE', #41246, #29996, #45373, .T. ) ;
#16475=EDGE_CURVE ( 'NONE', #20164, #12460, #33349, .T. ) ;
#16490=ORIENTED_EDGE ( 'NONE', *, *, #31148, .F. ) ;
#16501=EDGE_CURVE ( 'NONE', #18880, #7001, #41679, .T. ) ;
#16508=EDGE_CURVE ( 'NONE', #14904, #24881, #24552, .T. ) ;
#16512=DIRECTION ( 'NONE',  ( -1.000000000000000000, 0.000000000000000000, 0.000000000000000000 ) ) ;
#16521=EDGE_CURVE ( 'NONE', #27562, #2204, #2874, .T. ) ;
#16522=CYLINDRICAL_SURFACE ( 'NONE', #20237, 2.749999999999863665 ) ;
#16536=LINE ( 'NONE', #19530, #5417 ) ;
#16554=CARTESIAN_POINT ( 'NONE',  ( -598.8365100919716042, 256.5000000000001705, -202.7499999999898819 ) ) ;
#16583=VERTEX_POINT ( 'NONE', #28032 ) ;
#16593=AXIS2_PLACEMENT_3D ( 'NONE', #44011, #21935, #1971 ) ;
#16600=AXIS2_PLACEMENT_3D ( 'NONE', #33554, #40942, #16227 ) ;
#16628=CARTESIAN_POINT ( 'NONE',  ( -78.83651009197140525, 260.0000000000000568, -199.9999999999936051 ) ) ;
#16634=CIRCLE ( 'NONE', #3352, 2.749999999999835687 ) ;
#16650=ORIENTED_EDGE ( 'NONE', *, *, #39938, .T. ) ;
#16670=VERTEX_POINT ( 'NONE', #35196 ) ;
#16680=EDGE_CURVE ( 'NONE', #17388, #2565, #44917, .T. ) ;
#16685=AXIS2_PLACEMENT_3D ( 'NONE', #29353, #15027, #11568 ) ;
#16736=DIRECTION ( 'NONE',  ( -0.000000000000000000, 1.000000000000000000, -0.000000000000000000 ) ) ;
#16745=AXIS2_PLACEMENT_3D ( 'NONE', #27186, #41276, #44045 ) ;
#16773=AXIS2_PLACEMENT_3D ( 'NONE', #13051, #2187, #26889 ) ;
#16797=DIRECTION ( 'NONE',  ( -0.000000000000000000, 1.000000000000000000, -0.000000000000000000 ) ) ;
#16798=CARTESIAN_POINT ( 'NONE',  ( 181.1634899080285948, 260.0000000000000000, -193.8809999999953959 ) ) ;
#16803=ORIENTED_EDGE ( 'NONE', *, *, #23804, .F. ) ;
#16806=ADVANCED_FACE ( 'NONE', ( #39599, #21790 ), #42814, .F. ) ;
#16812=CARTESIAN_POINT ( 'NONE',  ( 701.1634899080286232, 259.9999999999999432, -199.9999999999990337 ) ) ;
#16836=VERTEX_POINT ( 'NONE', #31944 ) ;
#16837=ORIENTED_EDGE ( 'NONE', *, *, #35586, .T. ) ;
#16848=VECTOR ( 'NONE', #4539, 1000.000000000000000 ) ;
#16850=DIRECTION ( 'NONE',  ( 1.880165489482579047E-16, 1.000000000000000000, 0.000000000000000000 ) ) ;
#16853=CARTESIAN_POINT ( 'NONE',  ( 879.9999999999992042, 239.9999999999998863, -219.9999999999999716 ) ) ;
#16911=CARTESIAN_POINT ( 'NONE',  ( 181.1634899080285948, 256.5000000000000000, -206.1189999999954239 ) ) ;
#16942=AXIS2_PLACEMENT_3D ( 'NONE', #24321, #6089, #41666 ) ;
#16943=VERTEX_POINT ( 'NONE', #14419 ) ;
#16948=ORIENTED_EDGE ( 'NONE', *, *, #18978, .T. ) ;
#16966=DIRECTION ( 'NONE',  ( 1.000000000000000000, -1.892425610156518354E-16, 0.000000000000000000 ) ) ;
#17010=EDGE_CURVE ( 'NONE', #42674, #29342, #20752, .T. ) ;
#17016=CARTESIAN_POINT ( 'NONE',  ( -468.8365100919714337, 260.0000000000001705, -199.9999999999908766 ) ) ;
#17028=CARTESIAN_POINT ( 'NONE',  ( -598.8365100919716042, 240.0000000000001705, -199.9999999999899671 ) ) ;
#17070=DIRECTION ( 'NONE',  ( 0.000000000000000000, 0.000000000000000000, 1.000000000000000000 ) ) ;
#17090=DIRECTION ( 'NONE',  ( -0.000000000000000000, 1.000000000000000000, -0.000000000000000000 ) ) ;
#17107=DIRECTION ( 'NONE',  ( -0.000000000000000000, 1.000000000000000000, -0.000000000000000000 ) ) ;
#17142=DIRECTION ( 'NONE',  ( 0.000000000000000000, 0.000000000000000000, 1.000000000000000000 ) ) ;
#17165=ORIENTED_EDGE ( 'NONE', *, *, #28572, .T. ) ;
#17197=CARTESIAN_POINT ( 'NONE',  ( -338.8365100919713200, 240.0000000000001137, -202.7499999999916724 ) ) ;
#17243=CARTESIAN_POINT ( 'NONE',  ( 447.2824899080285945, 256.4999999999999432, -199.9999999999972431 ) ) ;
#17337=EDGE_CURVE ( 'NONE', #2204, #42341, #14911, .T. ) ;
#17339=AXIS2_PLACEMENT_3D ( 'NONE', #6506, #26655, #27971 ) ;
#17350=CIRCLE ( 'NONE', #9961, 8.025000000000003908 ) ;
#17355=VECTOR ( 'NONE', #21440, 1000.000000000000000 ) ;
#17388=VERTEX_POINT ( 'NONE', #16911 ) ;
#17404=EDGE_LOOP ( 'NONE', ( #30452, #30057 ) ) ;
#17420=DIRECTION ( 'NONE',  ( -0.000000000000000000, 1.000000000000000000, -0.000000000000000000 ) ) ;
#17422=ORIENTED_EDGE ( 'NONE', *, *, #1848, .F. ) ;
#17467=ORIENTED_EDGE ( 'NONE', *, *, #36014, .F. ) ;
#17484=FACE_OUTER_BOUND ( 'NONE', #3662, .T. ) ;
#17520=EDGE_CURVE ( 'NONE', #35282, #32688, #34801, .T. ) ;
#17553=CARTESIAN_POINT ( 'NONE',  ( 831.1634899080286232, 256.4999999999998863, -202.7499999999998863 ) ) ;
#17582=ORIENTED_EDGE ( 'NONE', *, *, #43051, .T. ) ;
#17602=AXIS2_PLACEMENT_3D ( 'NONE', #40345, #9530, #41176 ) ;
#17617=CARTESIAN_POINT ( 'NONE',  ( 181.1634899080285948, 260.0000000000000000, -199.9999999999953957 ) ) ;
#17635=( LENGTH_UNIT ( ) NAMED_UNIT ( * ) SI_UNIT ( .MILLI., .METRE. ) );
#17638=ORIENTED_EDGE ( 'NONE', *, *, #521, .F. ) ;
#17652=CARTESIAN_POINT ( 'NONE',  ( 701.1634899080286232, 259.9999999999999432, -199.9999999999990337 ) ) ;
#17657=CARTESIAN_POINT ( 'NONE',  ( 311.1634899080286232, 256.5000000000000000, -202.7499999999962483 ) ) ;
#17665=FACE_OUTER_BOUND ( 'NONE', #22321, .T. ) ;
#17699=EDGE_LOOP ( 'NONE', ( #10407, #18497, #1687, #27644 ) ) ;
#17707=VERTEX_POINT ( 'NONE', #14356 ) ;
#17728=FACE_OUTER_BOUND ( 'NONE', #20050, .T. ) ;
#17737=EDGE_LOOP ( 'NONE', ( #22280, #24090 ) ) ;
#17766=DIRECTION ( 'NONE',  ( 0.000000000000000000, 0.000000000000000000, 1.000000000000000000 ) ) ;
#17778=DIRECTION ( 'NONE',  ( 1.892425610156518354E-16, 1.000000000000000000, -0.000000000000000000 ) ) ;
#17811=CARTESIAN_POINT ( 'NONE',  ( -78.83651009197140525, 260.0000000000000568, -191.9749999999935994 ) ) ;
#17833=DIRECTION ( 'NONE',  ( -0.000000000000000000, 1.000000000000000000, -0.000000000000000000 ) ) ;
#17850=DIRECTION ( 'NONE',  ( 0.000000000000000000, 0.000000000000000000, 1.000000000000000000 ) ) ;
#17851=ORIENTED_EDGE ( 'NONE', *, *, #2980, .T. ) ;
#17858=ORIENTED_EDGE ( 'NONE', *, *, #34797, .F. ) ;
#17860=VERTEX_POINT ( 'NONE', #8334 ) ;
#17865=CARTESIAN_POINT ( 'NONE',  ( -468.8365100919714337, 260.0000000000001705, -199.9999999999908766 ) ) ;
#17880=EDGE_CURVE ( 'NONE', #10740, #12298, #44361, .T. ) ;
#17921=DIRECTION ( 'NONE',  ( -0.000000000000000000, 1.000000000000000000, -0.000000000000000000 ) ) ;
#17922=CARTESIAN_POINT ( 'NONE',  ( 441.1634899080286232, 256.4999999999999432, -199.9999999999972431 ) ) ;
#17928=AXIS2_PLACEMENT_3D ( 'NONE', #35942, #36168, #4310 ) ;
#17933=CARTESIAN_POINT ( 'NONE',  ( -208.8365100919714052, 260.0000000000001137, -208.0249999999927013 ) ) ;
#17935=CARTESIAN_POINT ( 'NONE',  ( 701.1634899080286232, 258.0939999999999372, -199.9999999999990337 ) ) ;
#17939=EDGE_CURVE ( 'NONE', #16583, #5387, #23074, .T. ) ;
#17943=FACE_OUTER_BOUND ( 'NONE', #38028, .T. ) ;
#17953=EDGE_CURVE ( 'NONE', #28279, #10881, #25438, .T. ) ;
#17975=EDGE_CURVE ( 'NONE', #36773, #41197, #3327, .T. ) ;
#17979=EDGE_CURVE ( 'NONE', #7749, #24881, #40186, .T. ) ;
#17994=VERTEX_POINT ( 'NONE', #33722 ) ;
#17997=CIRCLE ( 'NONE', #35680, 6.119000000000013095 ) ;
#18000=FACE_OUTER_BOUND ( 'NONE', #19138, .T. ) ;
#18025=CARTESIAN_POINT ( 'NONE',  ( -858.8365100919713768, 258.0940000000002215, -206.1189999999881479 ) ) ;
#18034=ORIENTED_EDGE ( 'NONE', *, *, #90, .F. ) ;
#18036=VECTOR ( 'NONE', #3182, 1000.000000000000000 ) ;
#18039=DIRECTION ( 'NONE',  ( 0.000000000000000000, 0.000000000000000000, 1.000000000000000000 ) ) ;
#18064=CARTESIAN_POINT ( 'NONE',  ( -208.8365100919714052, 256.5000000000001137, -199.9999999999926956 ) ) ;
#18073=VERTEX_POINT ( 'NONE', #18966 ) ;
#18076=CONICAL_SURFACE ( 'NONE', #45377, 8.025000000000003908, 0.7853981633974446153 ) ;
#18082=EDGE_LOOP ( 'NONE', ( #19481, #31200, #17165, #5259 ) ) ;
#18088=AXIS2_PLACEMENT_3D ( 'NONE', #25436, #509, #4216 ) ;
#18093=ADVANCED_FACE ( 'NONE', ( #12255 ), #32101, .F. ) ;
#18098=AXIS2_PLACEMENT_3D ( 'NONE', #19406, #36508, #8577 ) ;
#18102=ORIENTED_EDGE ( 'NONE', *, *, #25259, .T. ) ;
#18108=CIRCLE ( 'NONE', #7018, 6.118999999999985562 ) ;
#18115=AXIS2_PLACEMENT_3D ( 'NONE', #4033, #7505, #11192 ) ;
#18116=EDGE_CURVE ( 'NONE', #29342, #42674, #5549, .T. ) ;
#18128=CIRCLE ( 'NONE', #6304, 2.749999999999919176 ) ;
#18143=EDGE_CURVE ( 'NONE', #28937, #35282, #30245, .T. ) ;
#18178=CARTESIAN_POINT ( 'NONE',  ( -338.8365100919713200, 260.0000000000001137, -208.0249999999917918 ) ) ;
#18189=CIRCLE ( 'NONE', #35875, 2.749999999999891642 ) ;
#18190=DIRECTION ( 'NONE',  ( -0.000000000000000000, 1.000000000000000000, -0.000000000000000000 ) ) ;
#18191=LINE ( 'NONE', #18413, #16848 ) ;
#18207=AXIS2_PLACEMENT_3D ( 'NONE', #33257, #10949, #15700 ) ;
#18214=ORIENTED_EDGE ( 'NONE', *, *, #3549, .T. ) ;
#18215=PRODUCT_CONTEXT ( 'NONE', #4845, 'mechanical' ) ;
#18226=EDGE_CURVE ( 'NONE', #36701, #22122, #12931, .T. ) ;
#18248=DIRECTION ( 'NONE',  ( -0.000000000000000000, 1.000000000000000000, -0.000000000000000000 ) ) ;
#18250=AXIS2_PLACEMENT_3D ( 'NONE', #15539, #8616, #30073 ) ;
#18251=ADVANCED_FACE ( 'NONE', ( #10540 ), #24616, .F. ) ;
#18268=EDGE_CURVE ( 'NONE', #33524, #44027, #9258, .T. ) ;
#18281=VERTEX_POINT ( 'NONE', #41339 ) ;
#18302=FACE_OUTER_BOUND ( 'NONE', #40600, .T. ) ;
#18316=AXIS2_PLACEMENT_3D ( 'NONE', #25454, #21762, #64 ) ;
#18325=DIRECTION ( 'NONE',  ( -0.000000000000000000, 1.000000000000000000, -0.000000000000000000 ) ) ;
#18326=ORIENTED_EDGE ( 'NONE', *, *, #28143, .T. ) ;
#18328=VERTEX_POINT ( 'NONE', #156 ) ;
#18371=VERTEX_POINT ( 'NONE', #20307 ) ;
#18376=ORIENTED_EDGE ( 'NONE', *, *, #36838, .F. ) ;
#18399=LINE ( 'NONE', #11693, #32979 ) ;
#18402=CARTESIAN_POINT ( 'NONE',  ( 701.1634899080286232, 259.9999999999999432, -193.8809999999990623 ) ) ;
#18413=CARTESIAN_POINT ( 'NONE',  ( 181.1634899080285948, 260.0000000000000000, -202.7499999999952536 ) ) ;
#18427=VERTEX_POINT ( 'NONE', #28314 ) ;
#18472=EDGE_LOOP ( 'NONE', ( #33693, #28426, #22247, #20631 ) ) ;
#18479=ADVANCED_FACE ( 'NONE', ( #28786 ), #3844, .F. ) ;
#18488=EDGE_CURVE ( 'NONE', #38048, #39281, #18108, .T. ) ;
#18497=ORIENTED_EDGE ( 'NONE', *, *, #33183, .T. ) ;
#18501=CARTESIAN_POINT ( 'NONE',  ( 181.1634899080285948, 260.0000000000000000, -208.0249999999954014 ) ) ;
#18568=EDGE_CURVE ( 'NONE', #22786, #25461, #18399, .T. ) ;
#18610=ORIENTED_EDGE ( 'NONE', *, *, #39960, .T. ) ;
#18623=AXIS2_PLACEMENT_3D ( 'NONE', #26324, #19173, #39765 ) ;
#18625=DIRECTION ( 'NONE',  ( -0.000000000000000000, 1.000000000000000000, -0.000000000000000000 ) ) ;
#18653=EDGE_LOOP ( 'NONE', ( #5971, #4007, #6005, #38819 ) ) ;
#18665=DIRECTION ( 'NONE',  ( 0.000000000000000000, 0.000000000000000000, 1.000000000000000000 ) ) ;
#18681=EDGE_CURVE ( 'NONE', #3140, #25461, #24714, .T. ) ;
#18683=CIRCLE ( 'NONE', #17928, 2.749999999999919176 ) ;
#18756=EDGE_CURVE ( 'NONE', #14400, #29759, #32075, .T. ) ;
#18764=EDGE_LOOP ( 'NONE', ( #7456, #25575 ) ) ;
#18789=ADVANCED_FACE ( 'NONE', ( #25543 ), #19071, .F. ) ;
#18796=CARTESIAN_POINT ( 'NONE',  ( 181.1634899080285948, 260.0000000000000000, -199.9999999999953957 ) ) ;
#18798=CONICAL_SURFACE ( 'NONE', #28374, 8.025000000000003908, 0.7853981633974446153 ) ;
#18810=CARTESIAN_POINT ( 'NONE',  ( -338.8365100919713200, 258.0940000000001078, -206.1189999999917859 ) ) ;
#18812=CARTESIAN_POINT ( 'NONE',  ( -468.8365100919714337, 260.0000000000001705, -191.9749999999908709 ) ) ;
#18816=ADVANCED_FACE ( 'NONE', ( #1051 ), #18076, .F. ) ;
#18830=ORIENTED_EDGE ( 'NONE', *, *, #41132, .F. ) ;
#18838=LINE ( 'NONE', #136, #3391 ) ;
#18880=VERTEX_POINT ( 'NONE', #38599 ) ;
#18902=CIRCLE ( 'NONE', #4168, 8.024999999999948841 ) ;
#18908=CARTESIAN_POINT ( 'NONE',  ( -208.8365100919714052, 240.0000000000000853, -199.9999999999926956 ) ) ;
#18912=EDGE_LOOP ( 'NONE', ( #32560, #30008, #6024, #3299 ) ) ;
#18915=DIRECTION ( 'NONE',  ( -0.000000000000000000, 1.000000000000000000, -0.000000000000000000 ) ) ;
#18925=DIRECTION ( 'NONE',  ( -1.880165489482579047E-16, -1.000000000000000000, -0.000000000000000000 ) ) ;
#18966=CARTESIAN_POINT ( 'NONE',  ( -338.8365100919713200, 240.0000000000001137, -197.2499999999919282 ) ) ;
#18969=AXIS2_PLACEMENT_3D ( 'NONE', #33653, #19794, #16101 ) ;
#18978=EDGE_CURVE ( 'NONE', #15586, #27126, #21024, .T. ) ;
#18992=CARTESIAN_POINT ( 'NONE',  ( -598.8365100919716042, 260.0000000000001705, -199.9999999999899671 ) ) ;
#18993=ORIENTED_EDGE ( 'NONE', *, *, #1284, .T. ) ;
#19000=ORIENTED_EDGE ( 'NONE', *, *, #1578, .F. ) ;
#19011=ORIENTED_EDGE ( 'NONE', *, *, #25000, .T. ) ;
#19029=ADVANCED_FACE ( 'NONE', ( #37287 ), #1119, .F. ) ;
#19036=DIRECTION ( 'NONE',  ( 0.000000000000000000, 0.000000000000000000, 1.000000000000000000 ) ) ;
#19042=LINE ( 'NONE', #43729, #38179 ) ;
#19047=ORIENTED_EDGE ( 'NONE', *, *, #9197, .T. ) ;
#19053=ORIENTED_EDGE ( 'NONE', *, *, #31446, .F. ) ;
#19071=CYLINDRICAL_SURFACE ( 'NONE', #4816, 6.118999999999985562 ) ;
#19096=EDGE_LOOP ( 'NONE', ( #33253, #530, #14267, #24315 ) ) ;
#19100=DIRECTION ( 'NONE',  ( 0.000000000000000000, -0.000000000000000000, -1.000000000000000000 ) ) ;
#19109=ORIENTED_EDGE ( 'NONE', *, *, #25259, .F. ) ;
#19138=EDGE_LOOP ( 'NONE', ( #35677, #31592 ) ) ;
#19143=DIRECTION ( 'NONE',  ( -0.000000000000000000, 1.000000000000000000, -0.000000000000000000 ) ) ;
#19145=ORIENTED_EDGE ( 'NONE', *, *, #20363, .F. ) ;
#19158=ORIENTED_EDGE ( 'NONE', *, *, #23218, .T. ) ;
#19173=DIRECTION ( 'NONE',  ( -0.000000000000000000, 1.000000000000000000, -0.000000000000000000 ) ) ;
#19182=DIRECTION ( 'NONE',  ( -0.000000000000000000, 1.000000000000000000, -0.000000000000000000 ) ) ;
#19205=EDGE_LOOP ( 'NONE', ( #958, #43430, #13636, #3562 ) ) ;
#19213=ORIENTED_EDGE ( 'NONE', *, *, #39584, .F. ) ;
#19216=ORIENTED_EDGE ( 'NONE', *, *, #4150, .F. ) ;
#19245=CARTESIAN_POINT ( 'NONE',  ( 879.9999999999992042, 259.9999999999998863, -219.9999999999999716 ) ) ;
#19253=EDGE_LOOP ( 'NONE', ( #1527, #7244, #20300, #7482 ) ) ;
#19269=ORIENTED_EDGE ( 'NONE', *, *, #27224, .F. ) ;
#19271=CYLINDRICAL_SURFACE ( 'NONE', #10080, 6.118999999999985562 ) ;
#19275=CARTESIAN_POINT ( 'NONE',  ( -858.8365100919713768, 260.0000000000002274, -197.2499999999882903 ) ) ;
#19278=CARTESIAN_POINT ( 'NONE',  ( -338.8365100919713200, 256.5000000000001137, -199.9999999999917861 ) ) ;
#19310=DIRECTION ( 'NONE',  ( -0.000000000000000000, 1.000000000000000000, -0.000000000000000000 ) ) ;
#19344=EDGE_CURVE ( 'NONE', #12174, #16670, #15852, .T. ) ;
#19382=VERTEX_POINT ( 'NONE', #3161 ) ;
#19387=DIRECTION ( 'NONE',  ( -0.000000000000000000, 1.000000000000000000, -0.000000000000000000 ) ) ;
#19406=CARTESIAN_POINT ( 'NONE',  ( 701.1634899080286232, 239.9999999999999147, -199.9999999999990337 ) ) ;
#19407=DIRECTION ( 'NONE',  ( 0.000000000000000000, 0.000000000000000000, 1.000000000000000000 ) ) ;
#19435=ORIENTED_EDGE ( 'NONE', *, *, #18568, .F. ) ;
#19439=FACE_BOUND ( 'NONE', #41607, .T. ) ;
#19445=DIRECTION ( 'NONE',  ( -0.000000000000000000, 1.000000000000000000, -0.000000000000000000 ) ) ;
#19466=DIRECTION ( 'NONE',  ( -0.000000000000000000, 1.000000000000000000, -0.000000000000000000 ) ) ;
#19481=ORIENTED_EDGE ( 'NONE', *, *, #13445, .F. ) ;
#19503=DIRECTION ( 'NONE',  ( -0.000000000000000000, 1.000000000000000000, -0.000000000000000000 ) ) ;
#19530=CARTESIAN_POINT ( 'NONE',  ( 441.1634899080286232, 259.9999999999999432, -206.1189999999972144 ) ) ;
#19533=AXIS2_PLACEMENT_3D ( 'NONE', #168, #14040, #21190 ) ;
#19593=AXIS2_PLACEMENT_3D ( 'NONE', #17016, #6838, #41736 ) ;
#19628=DIRECTION ( 'NONE',  ( 0.000000000000000000, 0.000000000000000000, 1.000000000000000000 ) ) ;
#19635=DIRECTION ( 'NONE',  ( 0.000000000000000000, 0.000000000000000000, 1.000000000000000000 ) ) ;
#19690=AXIS2_PLACEMENT_3D ( 'NONE', #442, #28845, #4148 ) ;
#19707=EDGE_LOOP ( 'NONE', ( #16088, #42794, #21819, #4241 ) ) ;
#19720=ORIENTED_EDGE ( 'NONE', *, *, #7197, .F. ) ;
#19722=ORIENTED_EDGE ( 'NONE', *, *, #2930, .T. ) ;
#19728=DIRECTION ( 'NONE',  ( 0.000000000000000000, 0.000000000000000000, 1.000000000000000000 ) ) ;
#19733=CARTESIAN_POINT ( 'NONE',  ( -338.8365100919713200, 260.0000000000001137, -208.0249999999917918 ) ) ;
#19743=DIRECTION ( 'NONE',  ( -0.000000000000000000, 1.000000000000000000, -0.000000000000000000 ) ) ;
#19747=CARTESIAN_POINT ( 'NONE',  ( -338.8365100919713200, 260.0000000000001137, -206.1189999999917859 ) ) ;
#19794=DIRECTION ( 'NONE',  ( -0.000000000000000000, 1.000000000000000000, -0.000000000000000000 ) ) ;
#19848=EDGE_CURVE ( 'NONE', #31800, #27295, #27052, .T. ) ;
#19859=DIRECTION ( 'NONE',  ( 0.000000000000000000, 0.7071067811865474617, 0.7071067811865474617 ) ) ;
#19865=DIRECTION ( 'NONE',  ( -0.000000000000000000, 1.000000000000000000, -0.000000000000000000 ) ) ;
#19866=EDGE_CURVE ( 'NONE', #7749, #20164, #28320, .T. ) ;
#19870=ADVANCED_FACE ( 'NONE', ( #17728 ), #391, .F. ) ;
#19888=ORIENTED_EDGE ( 'NONE', *, *, #34286, .F. ) ;
#19898=ORIENTED_EDGE ( 'NONE', *, *, #8622, .F. ) ;
#19907=EDGE_CURVE ( 'NONE', #17994, #10694, #14940, .T. ) ;
#19948=EDGE_CURVE ( 'NONE', #35726, #14468, #24643, .T. ) ;
#20021=DIRECTION ( 'NONE',  ( 0.000000000000000000, 0.000000000000000000, 1.000000000000000000 ) ) ;
#20050=EDGE_LOOP ( 'NONE', ( #1322, #10647, #21639, #10936 ) ) ;
#20082=AXIS2_PLACEMENT_3D ( 'NONE', #42017, #38785, #10593 ) ;
#20088=DIRECTION ( 'NONE',  ( 0.000000000000000000, 0.000000000000000000, 1.000000000000000000 ) ) ;
#20105=DIRECTION ( 'NONE',  ( 0.000000000000000000, 0.000000000000000000, 1.000000000000000000 ) ) ;
#20111=EDGE_CURVE ( 'NONE', #21203, #4574, #12138, .T. ) ;
#20126=CYLINDRICAL_SURFACE ( 'NONE', #5682, 6.118999999999985562 ) ;
#20131=DIRECTION ( 'NONE',  ( 0.000000000000000000, 0.000000000000000000, 1.000000000000000000 ) ) ;
#20154=EDGE_CURVE ( 'NONE', #45239, #32411, #15111, .T. ) ;
#20164=VERTEX_POINT ( 'NONE', #4760 ) ;
#20172=EDGE_CURVE ( 'NONE', #12019, #9099, #5207, .T. ) ;
#20175=DIRECTION ( 'NONE',  ( -0.000000000000000000, 1.000000000000000000, -0.000000000000000000 ) ) ;
#20197=CARTESIAN_POINT ( 'NONE',  ( 311.1634899080286232, 258.0939999999999941, -199.9999999999963336 ) ) ;
#20206=EDGE_CURVE ( 'NONE', #4574, #30680, #40770, .T. ) ;
#20219=DIRECTION ( 'NONE',  ( 0.000000000000000000, 0.000000000000000000, 1.000000000000000000 ) ) ;
#20237=AXIS2_PLACEMENT_3D ( 'NONE', #23435, #27590, #5666 ) ;
#20259=ORIENTED_EDGE ( 'NONE', *, *, #17939, .T. ) ;
#20293=LINE ( 'NONE', #30010, #28486 ) ;
#20296=CARTESIAN_POINT ( 'NONE',  ( -598.8365100919716042, 256.5000000000001705, -199.9999999999899671 ) ) ;
#20300=ORIENTED_EDGE ( 'NONE', *, *, #36217, .T. ) ;
#20307=CARTESIAN_POINT ( 'NONE',  ( -468.8365100919714337, 260.0000000000001705, -208.0249999999908823 ) ) ;
#20337=ORIENTED_EDGE ( 'NONE', *, *, #42169, .T. ) ;
#20358=CIRCLE ( 'NONE', #5621, 2.749999999999891642 ) ;
#20363=EDGE_CURVE ( 'NONE', #29759, #10815, #8232, .T. ) ;
#20364=CIRCLE ( 'NONE', #27753, 6.118999999999985562 ) ;
#20384=AXIS2_PLACEMENT_3D ( 'NONE', #8437, #40535, #22740 ) ;
#20400=ORIENTED_EDGE ( 'NONE', *, *, #41017, .F. ) ;
#20405=CARTESIAN_POINT ( 'NONE',  ( 441.1634899080286232, 259.9999999999999432, -199.9999999999972431 ) ) ;
#20408=EDGE_LOOP ( 'NONE', ( #299, #31697, #8294, #4237 ) ) ;
#20411=DIRECTION ( 'NONE',  ( -0.000000000000000000, 1.000000000000000000, -0.000000000000000000 ) ) ;
#20421=LINE ( 'NONE', #44918, #31915 ) ;
#20457=VECTOR ( 'NONE', #33834, 1000.000000000000000 ) ;
#20481=CYLINDRICAL_SURFACE ( 'NONE', #7904, 6.118999999999985562 ) ;
#20487=EDGE_CURVE ( 'NONE', #12435, #27745, #20951, .T. ) ;
#20515=LINE ( 'NONE', #14051, #2521 ) ;
#20543=CARTESIAN_POINT ( 'NONE',  ( 311.1634899080286232, 258.0939999999999941, -206.1189999999963050 ) ) ;
#20558=AXIS2_PLACEMENT_3D ( 'NONE', #7334, #21410, #32719 ) ;
#20582=ORIENTED_EDGE ( 'NONE', *, *, #25473, .T. ) ;
#20599=FACE_OUTER_BOUND ( 'NONE', #19205, .T. ) ;
#20609=ORIENTED_EDGE ( 'NONE', *, *, #39725, .T. ) ;
#20615=CARTESIAN_POINT ( 'NONE',  ( 441.1634899080286232, 239.9999999999999716, -199.9999999999972431 ) ) ;
#20631=ORIENTED_EDGE ( 'NONE', *, *, #24693, .F. ) ;
#20637=DIRECTION ( 'NONE',  ( 0.000000000000000000, 0.000000000000000000, 1.000000000000000000 ) ) ;
#20640=DIRECTION ( 'NONE',  ( -0.000000000000000000, 1.000000000000000000, -0.000000000000000000 ) ) ;
#20643=ADVANCED_FACE ( 'NONE', ( #44463 ), #16522, .F. ) ;
#20660=DIRECTION ( 'NONE',  ( -0.000000000000000000, 1.000000000000000000, -0.000000000000000000 ) ) ;
#20670=ORIENTED_EDGE ( 'NONE', *, *, #20988, .T. ) ;
#20679=VERTEX_POINT ( 'NONE', #17197 ) ;
#20687=ORIENTED_EDGE ( 'NONE', *, *, #42896, .T. ) ;
#20692=CARTESIAN_POINT ( 'NONE',  ( 571.1634899080285095, 259.9999999999999432, -193.8809999999981528 ) ) ;
#20698=DIRECTION ( 'NONE',  ( -1.880165489482579047E-16, -1.000000000000000000, -0.000000000000000000 ) ) ;
#20708=ORIENTED_EDGE ( 'NONE', *, *, #34245, .F. ) ;
#20743=ADVANCED_FACE ( 'NONE', ( #9814 ), #16289, .F. ) ;
#20752=CIRCLE ( 'NONE', #13386, 8.025000000000003908 ) ;
#20762=ADVANCED_FACE ( 'NONE', ( #38001, #6357 ), #38230, .F. ) ;
#20793=ORIENTED_EDGE ( 'NONE', *, *, #41855, .T. ) ;
#20808=AXIS2_PLACEMENT_3D ( 'NONE', #7770, #14712, #39418 ) ;
#20817=FACE_BOUND ( 'NONE', #3948, .T. ) ;
#20844=VECTOR ( 'NONE', #27574, 999.9999999999998863 ) ;
#20863=LINE ( 'NONE', #3334, #25329 ) ;
#20882=CARTESIAN_POINT ( 'NONE',  ( 51.16348990802859475, 260.0000000000000568, -199.9999999999945146 ) ) ;
#20884=CARTESIAN_POINT ( 'NONE',  ( 441.1634899080286232, 258.0939999999999372, -193.8809999999972433 ) ) ;
#20902=EDGE_LOOP ( 'NONE', ( #32338, #2052 ) ) ;
#20916=AXIS2_PLACEMENT_3D ( 'NONE', #6096, #16736, #30819 ) ;
#20917=DIRECTION ( 'NONE',  ( 0.000000000000000000, 0.000000000000000000, 1.000000000000000000 ) ) ;
#20949=AXIS2_PLACEMENT_3D ( 'NONE', #6436, #31360, #9885 ) ;
#20951=CIRCLE ( 'NONE', #39452, 2.749999999999919176 ) ;
#20971=CARTESIAN_POINT ( 'NONE',  ( -879.9999999999992042, 240.0000000000002274, -219.9999999999999716 ) ) ;
#20975=ADVANCED_FACE ( 'NONE', ( #102 ), #42826, .F. ) ;
#20980=AXIS2_PLACEMENT_3D ( 'NONE', #12028, #19182, #19628 ) ;
#20988=EDGE_CURVE ( 'NONE', #36028, #3140, #11187, .T. ) ;
#21009=EDGE_CURVE ( 'NONE', #14468, #44027, #25038, .T. ) ;
#21017=EDGE_LOOP ( 'NONE', ( #25355, #21197, #39100, #12606 ) ) ;
#21021=AXIS2_PLACEMENT_3D ( 'NONE', #5155, #43716, #43497 ) ;
#21024=CIRCLE ( 'NONE', #32846, 2.749999999999891642 ) ;
#21035=CIRCLE ( 'NONE', #26181, 6.118999999999985562 ) ;
#21044=VECTOR ( 'NONE', #25292, 999.9999999999998863 ) ;
#21063=DIRECTION ( 'NONE',  ( 0.000000000000000000, 0.000000000000000000, 1.000000000000000000 ) ) ;
#21079=ORIENTED_EDGE ( 'NONE', *, *, #16234, .T. ) ;
#21089=CIRCLE ( 'NONE', #33643, 2.749999999999863665 ) ;
#21136=AXIS2_PLACEMENT_3D ( 'NONE', #32357, #42963, #11331 ) ;
#21140=DIRECTION ( 'NONE',  ( -0.000000000000000000, 1.000000000000000000, -0.000000000000000000 ) ) ;
#21154=CIRCLE ( 'NONE', #2691, 6.118999999999985562 ) ;
#21158=ORIENTED_EDGE ( 'NONE', *, *, #30903, .T. ) ;
#21168=DIRECTION ( 'NONE',  ( -0.000000000000000000, 1.000000000000000000, -0.000000000000000000 ) ) ;
#21190=DIRECTION ( 'NONE',  ( 0.000000000000000000, 0.000000000000000000, 1.000000000000000000 ) ) ;
#21193=CIRCLE ( 'NONE', #33037, 2.749999999999863665 ) ;
#21197=ORIENTED_EDGE ( 'NONE', *, *, #28109, .F. ) ;
#21203=VERTEX_POINT ( 'NONE', #567 ) ;
#21215=ORIENTED_EDGE ( 'NONE', *, *, #1239, .T. ) ;
#21217=CARTESIAN_POINT ( 'NONE',  ( 831.1634899080286232, 259.9999999999998863, -206.1189999999999429 ) ) ;
#21229=CARTESIAN_POINT ( 'NONE',  ( 181.1634899080285948, 258.0939999999999941, -199.9999999999953957 ) ) ;
#21268=CARTESIAN_POINT ( 'NONE',  ( -338.8365100919713200, 256.5000000000001137, -202.7499999999917009 ) ) ;
#21321=VERTEX_POINT ( 'NONE', #43279 ) ;
#21327=DIRECTION ( 'NONE',  ( 0.000000000000000000, 0.000000000000000000, 1.000000000000000000 ) ) ;
#21328=ORIENTED_EDGE ( 'NONE', *, *, #1789, .F. ) ;
#21364=ADVANCED_FACE ( 'NONE', ( #25937, #29863 ), #22469, .F. ) ;
#21387=CYLINDRICAL_SURFACE ( 'NONE', #45429, 6.118999999999985562 ) ;
#21403=CARTESIAN_POINT ( 'NONE',  ( 701.1634899080286232, 256.4999999999999432, -206.1189999999990334 ) ) ;
#21410=DIRECTION ( 'NONE',  ( -0.000000000000000000, 1.000000000000000000, -0.000000000000000000 ) ) ;
#21415=CYLINDRICAL_SURFACE ( 'NONE', #33582, 6.119000000000013095 ) ;
#21427=ORIENTED_EDGE ( 'NONE', *, *, #10616, .T. ) ;
#21440=DIRECTION ( 'NONE',  ( -0.000000000000000000, 1.000000000000000000, -0.000000000000000000 ) ) ;
#21445=CARTESIAN_POINT ( 'NONE',  ( -728.8365100919714905, 260.0000000000001705, -193.8809999999890863 ) ) ;
#21453=DIRECTION ( 'NONE',  ( -0.000000000000000000, 1.000000000000000000, -0.000000000000000000 ) ) ;
#21531=DIRECTION ( 'NONE',  ( -1.000000000000000000, 0.000000000000000000, 0.000000000000000000 ) ) ;
#21570=EDGE_CURVE ( 'NONE', #25461, #3140, #3336, .T. ) ;
#21572=DIRECTION ( 'NONE',  ( 0.000000000000000000, 0.7071067811865578978, 0.7071067811865372477 ) ) ;
#21597=EDGE_CURVE ( 'NONE', #29996, #40012, #12890, .T. ) ;
#21604=CARTESIAN_POINT ( 'NONE',  ( 181.1634899080285948, 260.0000000000000000, -199.9999999999953957 ) ) ;
#21605=DIRECTION ( 'NONE',  ( 0.000000000000000000, 0.000000000000000000, 1.000000000000000000 ) ) ;
#21615=EDGE_CURVE ( 'NONE', #32511, #2565, #21756, .T. ) ;
#21639=ORIENTED_EDGE ( 'NONE', *, *, #39584, .T. ) ;
#21640=AXIS2_PLACEMENT_3D ( 'NONE', #37582, #15658, #12199 ) ;
#21653=EDGE_LOOP ( 'NONE', ( #35379, #21811, #30902, #5120 ) ) ;
#21667=CARTESIAN_POINT ( 'NONE',  ( -468.8365100919714337, 260.0000000000001705, -202.7499999999907345 ) ) ;
#21676=AXIS2_PLACEMENT_3D ( 'NONE', #33836, #37061, #9359 ) ;
#21688=DIRECTION ( 'NONE',  ( 0.000000000000000000, 0.000000000000000000, 1.000000000000000000 ) ) ;
#21716=AXIS2_PLACEMENT_3D ( 'NONE', #43401, #36461, #895 ) ;
#21717=DIRECTION ( 'NONE',  ( -0.000000000000000000, 1.000000000000000000, -0.000000000000000000 ) ) ;
#21723=VERTEX_POINT ( 'NONE', #25382 ) ;
#21756=CIRCLE ( 'NONE', #11449, 6.119000000000013095 ) ;
#21762=DIRECTION ( 'NONE',  ( -0.000000000000000000, 1.000000000000000000, -0.000000000000000000 ) ) ;
#21765=ORIENTED_EDGE ( 'NONE', *, *, #13710, .F. ) ;
#21768=AXIS2_PLACEMENT_3D ( 'NONE', #35371, #45563, #13457 ) ;
#21773=AXIS2_PLACEMENT_3D ( 'NONE', #678, #446, #43168 ) ;
#21790=FACE_OUTER_BOUND ( 'NONE', #1473, .T. ) ;
#21811=ORIENTED_EDGE ( 'NONE', *, *, #34823, .F. ) ;
#21819=ORIENTED_EDGE ( 'NONE', *, *, #17010, .T. ) ;
#21834=DIRECTION ( 'NONE',  ( 0.000000000000000000, -0.000000000000000000, -1.000000000000000000 ) ) ;
#21844=DIRECTION ( 'NONE',  ( -0.000000000000000000, 1.000000000000000000, -0.000000000000000000 ) ) ;
#21848=AXIS2_PLACEMENT_3D ( 'NONE', #34520, #10481, #23871 ) ;
#21850=DIRECTION ( 'NONE',  ( -1.000000000000000000, 1.892425610156518354E-16, 0.000000000000000000 ) ) ;
#21912=LINE ( 'NONE', #4579, #42561 ) ;
#21919=CIRCLE ( 'NONE', #33706, 8.024999999999948841 ) ;
#21924=CIRCLE ( 'NONE', #40363, 2.749999999999919176 ) ;
#21935=DIRECTION ( 'NONE',  ( -0.000000000000000000, 1.000000000000000000, -0.000000000000000000 ) ) ;
#21983=DIRECTION ( 'NONE',  ( 0.000000000000000000, 0.000000000000000000, 1.000000000000000000 ) ) ;
#21998=DIRECTION ( 'NONE',  ( 0.000000000000000000, 0.000000000000000000, 1.000000000000000000 ) ) ;
#22022=DIRECTION ( 'NONE',  ( 0.000000000000000000, 0.000000000000000000, 1.000000000000000000 ) ) ;
#22068=FACE_OUTER_BOUND ( 'NONE', #38837, .T. ) ;
#22071=CARTESIAN_POINT ( 'NONE',  ( -208.8365100919714052, 260.0000000000001137, -199.9999999999926956 ) ) ;
#22077=FACE_BOUND ( 'NONE', #30290, .T. ) ;
#22122=VERTEX_POINT ( 'NONE', #6582 ) ;
#22134=CARTESIAN_POINT ( 'NONE',  ( 441.1634899080286232, 259.9999999999999432, -208.0249999999972488 ) ) ;
#22151=FACE_OUTER_BOUND ( 'NONE', #37669, .T. ) ;
#22188=EDGE_CURVE ( 'NONE', #12298, #10740, #40978, .T. ) ;
#22211=FACE_OUTER_BOUND ( 'NONE', #27112, .T. ) ;
#22225=CARTESIAN_POINT ( 'NONE',  ( 51.16348990802859475, 260.0000000000000568, -191.9749999999945089 ) ) ;
#22247=ORIENTED_EDGE ( 'NONE', *, *, #19948, .T. ) ;
#22270=AXIS2_PLACEMENT_3D ( 'NONE', #33599, #30134, #41223 ) ;
#22280=ORIENTED_EDGE ( 'NONE', *, *, #34823, .T. ) ;
#22282=DIRECTION ( 'NONE',  ( 0.000000000000000000, 0.000000000000000000, 1.000000000000000000 ) ) ;
#22318=CIRCLE ( 'NONE', #29004, 2.749999999999863665 ) ;
#22321=EDGE_LOOP ( 'NONE', ( #39398, #33969, #33519, #33762 ) ) ;
#22338=DIRECTION ( 'NONE',  ( 0.000000000000000000, 0.000000000000000000, 1.000000000000000000 ) ) ;
#22362=FACE_OUTER_BOUND ( 'NONE', #4560, .T. ) ;
#22371=VERTEX_POINT ( 'NONE', #28518 ) ;
#22387=ADVANCED_FACE ( 'NONE', ( #42614 ), #334, .F. ) ;
#22428=AXIS2_PLACEMENT_3D ( 'NONE', #41312, #45006, #10342 ) ;
#22432=AXIS2_PLACEMENT_3D ( 'NONE', #43108, #4538, #31576 ) ;
#22451=FACE_OUTER_BOUND ( 'NONE', #13332, .T. ) ;
#22461=FACE_OUTER_BOUND ( 'NONE', #18082, .T. ) ;
#22469=PLANE ( 'NONE',  #21021 ) ;
#22471=ORIENTED_EDGE ( 'NONE', *, *, #2953, .F. ) ;
#22491=ORIENTED_EDGE ( 'NONE', *, *, #2744, .T. ) ;
#22502=FACE_OUTER_BOUND ( 'NONE', #29341, .T. ) ;
#22503=LINE ( 'NONE', #12122, #448 ) ;
#22516=DIRECTION ( 'NONE',  ( 1.892425610156518354E-16, 1.000000000000000000, -0.000000000000000000 ) ) ;
#22523=AXIS2_PLACEMENT_3D ( 'NONE', #34775, #41958, #6145 ) ;
#22538=ORIENTED_EDGE ( 'NONE', *, *, #4622, .T. ) ;
#22556=ORIENTED_EDGE ( 'NONE', *, *, #28976, .F. ) ;
#22574=LINE ( 'NONE', #11962, #30432 ) ;
#22604=ADVANCED_FACE ( 'NONE', ( #15117 ), #12957, .F. ) ;
#22607=VERTEX_POINT ( 'NONE', #18810 ) ;
#22623=CARTESIAN_POINT ( 'NONE',  ( -78.83651009197140525, 260.0000000000000568, -199.9999999999936051 ) ) ;
#22632=CIRCLE ( 'NONE', #26331, 8.025000000000003908 ) ;
#22639=CIRCLE ( 'NONE', #38151, 6.118999999999985562 ) ;
#22676=ORIENTED_EDGE ( 'NONE', *, *, #7494, .F. ) ;
#22701=EDGE_CURVE ( 'NONE', #14461, #40963, #36804, .T. ) ;
#22710=EDGE_LOOP ( 'NONE', ( #42580, #44261, #1432, #12074 ) ) ;
#22736=DIRECTION ( 'NONE',  ( -0.000000000000000000, 1.000000000000000000, -0.000000000000000000 ) ) ;
#22740=DIRECTION ( 'NONE',  ( 0.000000000000000000, 0.000000000000000000, 1.000000000000000000 ) ) ;
#22749=FACE_BOUND ( 'NONE', #7312, .T. ) ;
#22762=EDGE_CURVE ( 'NONE', #16836, #42559, #6288, .T. ) ;
#22772=ADVANCED_FACE ( 'NONE', ( #8857 ), #34313, .F. ) ;
#22778=ORIENTED_EDGE ( 'NONE', *, *, #9146, .T. ) ;
#22786=VERTEX_POINT ( 'NONE', #37485 ) ;
#22797=CONICAL_SURFACE ( 'NONE', #29441, 8.025000000000003908, 0.7853981633974410625 ) ;
#22802=CARTESIAN_POINT ( 'NONE',  ( -468.8365100919714337, 240.0000000000001421, -199.9999999999908766 ) ) ;
#22803=DIRECTION ( 'NONE',  ( 1.892425610156518354E-16, 1.000000000000000000, -0.000000000000000000 ) ) ;
#22852=VERTEX_POINT ( 'NONE', #40049 ) ;
#22884=CARTESIAN_POINT ( 'NONE',  ( -468.8365100919714337, 260.0000000000001705, -197.2499999999910187 ) ) ;
#22900=CARTESIAN_POINT ( 'NONE',  ( 311.1634899080286232, 260.0000000000000000, -197.2499999999964473 ) ) ;
#22949=CARTESIAN_POINT ( 'NONE',  ( -879.9999999999992042, 260.0000000000002274, -179.9999999999999716 ) ) ;
#22996=ORIENTED_EDGE ( 'NONE', *, *, #37891, .F. ) ;
#22998=ORIENTED_EDGE ( 'NONE', *, *, #2759, .T. ) ;
#23004=DIRECTION ( 'NONE',  ( -0.000000000000000000, 1.000000000000000000, -0.000000000000000000 ) ) ;
#23038=CARTESIAN_POINT ( 'NONE',  ( 571.1634899080285095, 259.9999999999999432, -199.9999999999981526 ) ) ;
#23044=DIRECTION ( 'NONE',  ( 8.659560562354807133E-17, 0.7071067811865578978, -0.7071067811865372477 ) ) ;
#23045=ORIENTED_EDGE ( 'NONE', *, *, #25473, .F. ) ;
#23048=EDGE_CURVE ( 'NONE', #44849, #39281, #6059, .T. ) ;
#23055=ORIENTED_EDGE ( 'NONE', *, *, #14023, .T. ) ;
#23074=LINE ( 'NONE', #4865, #29856 ) ;
#23080=DIRECTION ( 'NONE',  ( -0.000000000000000000, 1.000000000000000000, -0.000000000000000000 ) ) ;
#23106=ORIENTED_EDGE ( 'NONE', *, *, #42760, .F. ) ;
#23114=CARTESIAN_POINT ( 'NONE',  ( 51.16348990802859475, 240.0000000000000568, -199.9999999999945146 ) ) ;
#23125=DIRECTION ( 'NONE',  ( 0.000000000000000000, 0.000000000000000000, 1.000000000000000000 ) ) ;
#23143=ORIENTED_EDGE ( 'NONE', *, *, #12533, .F. ) ;
#23153=CARTESIAN_POINT ( 'NONE',  ( 0.000000000000000000, 0.000000000000000000, 0.000000000000000000 ) ) ;
#23156=AXIS2_PLACEMENT_3D ( 'NONE', #547, #42338, #3323 ) ;
#23157=ORIENTED_EDGE ( 'NONE', *, *, #39633, .F. ) ;
#23185=VECTOR ( 'NONE', #21572, 999.9999999999998863 ) ;
#23186=CARTESIAN_POINT ( 'NONE',  ( -598.8365100919716042, 256.5000000000001705, -199.9999999999899671 ) ) ;
#23189=CARTESIAN_POINT ( 'NONE',  ( -598.8365100919716042, 256.5000000000001705, -197.2499999999900524 ) ) ;
#23213=VECTOR ( 'NONE', #18925, 1000.000000000000000 ) ;
#23218=EDGE_CURVE ( 'NONE', #25919, #18880, #39521, .T. ) ;
#23224=EDGE_LOOP ( 'NONE', ( #37840, #28698 ) ) ;
#23226=VERTEX_POINT ( 'NONE', #3137 ) ;
#23242=DIRECTION ( 'NONE',  ( -0.000000000000000000, 1.000000000000000000, -0.000000000000000000 ) ) ;
#23273=DIRECTION ( 'NONE',  ( 0.000000000000000000, 0.000000000000000000, 1.000000000000000000 ) ) ;
#23285=ORIENTED_EDGE ( 'NONE', *, *, #29254, .F. ) ;
#23289=AXIS2_PLACEMENT_3D ( 'NONE', #28074, #30638, #38713 ) ;
#23305=ORIENTED_EDGE ( 'NONE', *, *, #14520, .T. ) ;
#23312=CARTESIAN_POINT ( 'NONE',  ( -78.83651009197140525, 256.5000000000000568, -199.9999999999936051 ) ) ;
#23358=AXIS2_PLACEMENT_3D ( 'NONE', #41043, #37105, #37346 ) ;
#23435=CARTESIAN_POINT ( 'NONE',  ( 571.1634899080285095, 259.9999999999999432, -199.9999999999981526 ) ) ;
#23471=CARTESIAN_POINT ( 'NONE',  ( 51.16348990802859475, 240.0000000000000568, -197.2499999999946851 ) ) ;
#23475=DIRECTION ( 'NONE',  ( -0.000000000000000000, 1.000000000000000000, -0.000000000000000000 ) ) ;
#23477=ORIENTED_EDGE ( 'NONE', *, *, #3549, .F. ) ;
#23508=CIRCLE ( 'NONE', #42002, 6.118999999999985562 ) ;
#23521=DIRECTION ( 'NONE',  ( 0.000000000000000000, 0.000000000000000000, 1.000000000000000000 ) ) ;
#23561=DIRECTION ( 'NONE',  ( -0.000000000000000000, 1.000000000000000000, -0.000000000000000000 ) ) ;
#23587=DIRECTION ( 'NONE',  ( 0.000000000000000000, 0.000000000000000000, 1.000000000000000000 ) ) ;
#23628=DIRECTION ( 'NONE',  ( 1.892425610156518354E-16, 1.000000000000000000, -0.000000000000000000 ) ) ;
#23633=ORIENTED_EDGE ( 'NONE', *, *, #43019, .F. ) ;
#23636=DIRECTION ( 'NONE',  ( -0.000000000000000000, 1.000000000000000000, -0.000000000000000000 ) ) ;
#23640=DIRECTION ( 'NONE',  ( 0.000000000000000000, 0.000000000000000000, 1.000000000000000000 ) ) ;
#23655=DIRECTION ( 'NONE',  ( 0.000000000000000000, -1.000000000000000000, 0.000000000000000000 ) ) ;
#23659=DIRECTION ( 'NONE',  ( -0.000000000000000000, 1.000000000000000000, -0.000000000000000000 ) ) ;
#23697=CARTESIAN_POINT ( 'NONE',  ( 701.1634899080286232, 256.4999999999999432, -199.9999999999990337 ) ) ;
#23726=LINE ( 'NONE', #24645, #18036 ) ;
#23737=CIRCLE ( 'NONE', #22270, 6.118999999999985562 ) ;
#23741=LINE ( 'NONE', #37852, #26274 ) ;
#23757=EDGE_CURVE ( 'NONE', #4574, #21203, #32145, .T. ) ;
#23793=AXIS2_PLACEMENT_3D ( 'NONE', #32253, #24855, #25080 ) ;
#23804=EDGE_CURVE ( 'NONE', #21321, #18281, #4842, .T. ) ;
#23811=DIRECTION ( 'NONE',  ( -0.000000000000000000, 1.000000000000000000, -0.000000000000000000 ) ) ;
#23852=LINE ( 'NONE', #34255, #34366 ) ;
#23867=DIRECTION ( 'NONE',  ( -0.000000000000000000, 1.000000000000000000, -0.000000000000000000 ) ) ;
#23871=DIRECTION ( 'NONE',  ( 0.000000000000000000, 0.000000000000000000, 1.000000000000000000 ) ) ;
#23895=AXIS2_PLACEMENT_3D ( 'NONE', #7434, #733, #35587 ) ;
#23915=VECTOR ( 'NONE', #12596, 1000.000000000000000 ) ;
#23921=CARTESIAN_POINT ( 'NONE',  ( 51.16348990802859475, 260.0000000000000568, -208.0249999999945203 ) ) ;
#23925=DIRECTION ( 'NONE',  ( 0.000000000000000000, 0.000000000000000000, 1.000000000000000000 ) ) ;
#23929=CIRCLE ( 'NONE', #12902, 6.118999999999985562 ) ;
#23938=ORIENTED_EDGE ( 'NONE', *, *, #34245, .T. ) ;
#23945=CARTESIAN_POINT ( 'NONE',  ( 51.16348990802859475, 256.5000000000000568, -206.1189999999945428 ) ) ;
#23955=AXIS2_PLACEMENT_3D ( 'NONE', #18064, #36072, #39311 ) ;
#23958=CIRCLE ( 'NONE', #30604, 6.119000000000013095 ) ;
#23960=ORIENTED_EDGE ( 'NONE', *, *, #36478, .T. ) ;
#23980=ORIENTED_EDGE ( 'NONE', *, *, #41132, .T. ) ;
#24028=ORIENTED_EDGE ( 'NONE', *, *, #32371, .F. ) ;
#24034=ORIENTED_EDGE ( 'NONE', *, *, #6043, .T. ) ;
#24039=AXIS2_PLACEMENT_3D ( 'NONE', #29755, #26055, #10442 ) ;
#24052=ADVANCED_FACE ( 'NONE', ( #15584 ), #8433, .F. ) ;
#24054=PLANE ( 'NONE',  #21768 ) ;
#24076=ADVANCED_FACE ( 'NONE', ( #22502 ), #40317, .F. ) ;
#24090=ORIENTED_EDGE ( 'NONE', *, *, #919, .T. ) ;
#24097=CIRCLE ( 'NONE', #16006, 6.119000000000013095 ) ;
#24103=DIRECTION ( 'NONE',  ( 0.000000000000000000, 0.000000000000000000, 1.000000000000000000 ) ) ;
#24106=ADVANCED_FACE ( 'NONE', ( #1275, #26643 ), #40739, .F. ) ;
#24121=ADVANCED_FACE ( 'NONE', ( #26430 ), #29892, .F. ) ;
#24122=DIRECTION ( 'NONE',  ( -0.000000000000000000, 1.000000000000000000, -0.000000000000000000 ) ) ;
#24177=EDGE_CURVE ( 'NONE', #41429, #37578, #10754, .T. ) ;
#24192=CARTESIAN_POINT ( 'NONE',  ( -728.8365100919714905, 256.5000000000001705, -197.2499999999891429 ) ) ;
#24211=AXIS2_PLACEMENT_3D ( 'NONE', #16812, #24397, #27642 ) ;
#24217=CARTESIAN_POINT ( 'NONE',  ( -208.8365100919714052, 260.0000000000001137, -199.9999999999926956 ) ) ;
#24286=CARTESIAN_POINT ( 'NONE',  ( -208.8365100919714052, 256.5000000000001137, -199.9999999999926956 ) ) ;
#24312=EDGE_LOOP ( 'NONE', ( #29659, #45110, #34821, #38463 ) ) ;
#24315=ORIENTED_EDGE ( 'NONE', *, *, #18116, .T. ) ;
#24321=CARTESIAN_POINT ( 'NONE',  ( -468.8365100919714337, 260.0000000000001705, -199.9999999999908766 ) ) ;
#24331=DIRECTION ( 'NONE',  ( 0.000000000000000000, 0.000000000000000000, 1.000000000000000000 ) ) ;
#24359=EDGE_LOOP ( 'NONE', ( #11730, #35107 ) ) ;
#24373=CARTESIAN_POINT ( 'NONE',  ( -78.83651009197140525, 260.0000000000000568, -208.0249999999936108 ) ) ;
#24375=EDGE_CURVE ( 'NONE', #17707, #5383, #38841, .T. ) ;
#24391=EDGE_CURVE ( 'NONE', #27295, #8740, #7193, .T. ) ;
#24392=DIRECTION ( 'NONE',  ( -0.000000000000000000, 1.000000000000000000, -0.000000000000000000 ) ) ;
#24397=DIRECTION ( 'NONE',  ( -0.000000000000000000, 1.000000000000000000, -0.000000000000000000 ) ) ;
#24405=CARTESIAN_POINT ( 'NONE',  ( -338.8365100919713200, 256.5000000000001137, -193.8809999999918148 ) ) ;
#24426=ADVANCED_FACE ( 'NONE', ( #43198 ), #43257, .F. ) ;
#24435=FACE_OUTER_BOUND ( 'NONE', #5174, .T. ) ;
#24443=AXIS2_PLACEMENT_3D ( 'NONE', #29581, #8791, #43657 ) ;
#24477=EDGE_CURVE ( 'NONE', #28297, #34711, #20364, .T. ) ;
#24509=FACE_BOUND ( 'NONE', #43316, .T. ) ;
#24526=CIRCLE ( 'NONE', #42217, 2.749999999999835687 ) ;
#24546=ORIENTED_EDGE ( 'NONE', *, *, #36196, .F. ) ;
#24552=LINE ( 'NONE', #38435, #25242 ) ;
#24599=EDGE_CURVE ( 'NONE', #2565, #18281, #4410, .T. ) ;
#24611=DIRECTION ( 'NONE',  ( -0.000000000000000000, 1.000000000000000000, -0.000000000000000000 ) ) ;
#24616=CYLINDRICAL_SURFACE ( 'NONE', #28405, 6.119000000000013095 ) ;
#24620=EDGE_CURVE ( 'NONE', #28279, #13947, #7640, .T. ) ;
#24621=DIRECTION ( 'NONE',  ( -0.000000000000000000, 1.000000000000000000, -0.000000000000000000 ) ) ;
#24625=CARTESIAN_POINT ( 'NONE',  ( -208.8365100919714052, 260.0000000000001137, -199.9999999999926956 ) ) ;
#24633=ORIENTED_EDGE ( 'NONE', *, *, #42896, .F. ) ;
#24639=ORIENTED_EDGE ( 'NONE', *, *, #37651, .T. ) ;
#24643=CIRCLE ( 'NONE', #8449, 6.118999999999985562 ) ;
#24645=CARTESIAN_POINT ( 'NONE',  ( -879.9999999999992042, 260.0000000000002274, -219.9999999999999716 ) ) ;
#24665=CARTESIAN_POINT ( 'NONE',  ( -338.8365100919713200, 260.0000000000001137, -191.9749999999917804 ) ) ;
#24666=DIRECTION ( 'NONE',  ( 0.000000000000000000, -0.000000000000000000, -1.000000000000000000 ) ) ;
#24678=EDGE_CURVE ( 'NONE', #30282, #22122, #32954, .T. ) ;
#24682=EDGE_CURVE ( 'NONE', #22852, #34024, #18189, .T. ) ;
#24684=CARTESIAN_POINT ( 'NONE',  ( -208.8365100919714052, 256.5000000000001137, -193.8809999999926674 ) ) ;
#24693=EDGE_CURVE ( 'NONE', #7627, #14468, #20293, .T. ) ;
#24695=MECHANICAL_DESIGN_GEOMETRIC_PRESENTATION_REPRESENTATION('',(#43147),#15831);
#24699=VECTOR ( 'NONE', #23811, 1000.000000000000000 ) ;
#24710=AXIS2_PLACEMENT_3D ( 'NONE', #24873, #14947, #29270 ) ;
#24714=CIRCLE ( 'NONE', #7759, 2.749999999999919176 ) ;
#24723=FACE_OUTER_BOUND ( 'NONE', #8882, .T. ) ;
#24728=CIRCLE ( 'NONE', #26941, 2.749999999999835687 ) ;
#24752=DIRECTION ( 'NONE',  ( -0.000000000000000000, 1.000000000000000000, -0.000000000000000000 ) ) ;
#24770=ORIENTED_EDGE ( 'NONE', *, *, #35122, .F. ) ;
#24810=DIRECTION ( 'NONE',  ( -0.000000000000000000, 1.000000000000000000, -0.000000000000000000 ) ) ;
#24818=ORIENTED_EDGE ( 'NONE', *, *, #21570, .F. ) ;
#24819=AXIS2_PLACEMENT_3D ( 'NONE', #45024, #34835, #41548 ) ;
#24848=CIRCLE ( 'NONE', #34183, 6.118999999999985562 ) ;
#24855=DIRECTION ( 'NONE',  ( -0.000000000000000000, 1.000000000000000000, -0.000000000000000000 ) ) ;
#24866=DIRECTION ( 'NONE',  ( -0.000000000000000000, 1.000000000000000000, -0.000000000000000000 ) ) ;
#24873=CARTESIAN_POINT ( 'NONE',  ( -338.8365100919713200, 260.0000000000001137, -199.9999999999917861 ) ) ;
#24881=VERTEX_POINT ( 'NONE', #41326 ) ;
#24899=CARTESIAN_POINT ( 'NONE',  ( -208.8365100919714052, 256.5000000000001137, -199.9999999999926956 ) ) ;
#24913=AXIS2_PLACEMENT_3D ( 'NONE', #14852, #18325, #43239 ) ;
#24980=CARTESIAN_POINT ( 'NONE',  ( -728.8365100919714905, 256.5000000000001705, -199.9999999999890861 ) ) ;
#25000=EDGE_CURVE ( 'NONE', #10586, #23226, #23741, .T. ) ;
#25015=ADVANCED_FACE ( 'NONE', ( #34385 ), #40865, .F. ) ;
#25021=CARTESIAN_POINT ( 'NONE',  ( -728.8365100919714905, 258.0940000000001646, -199.9999999999890861 ) ) ;
#25022=ORIENTED_EDGE ( 'NONE', *, *, #6020, .T. ) ;
#25038=LINE ( 'NONE', #14194, #23185 ) ;
#25052=CARTESIAN_POINT ( 'NONE',  ( -598.8365100919716042, 258.0940000000001646, -199.9999999999899671 ) ) ;
#25074=DIRECTION ( 'NONE',  ( -0.000000000000000000, 1.000000000000000000, -0.000000000000000000 ) ) ;
#25080=DIRECTION ( 'NONE',  ( 0.000000000000000000, 0.000000000000000000, 1.000000000000000000 ) ) ;
#25140=CARTESIAN_POINT ( 'NONE',  ( 701.1634899080286232, 258.0939999999999372, -199.9999999999990337 ) ) ;
#25144=FACE_OUTER_BOUND ( 'NONE', #11146, .T. ) ;
#25224=ORIENTED_EDGE ( 'NONE', *, *, #20487, .F. ) ;
#25228=ORIENTED_EDGE ( 'NONE', *, *, #20988, .F. ) ;
#25232=ADVANCED_FACE ( 'NONE', ( #7138 ), #31379, .F. ) ;
#25234=DIRECTION ( 'NONE',  ( -0.000000000000000000, 1.000000000000000000, -0.000000000000000000 ) ) ;
#25242=VECTOR ( 'NONE', #20640, 1000.000000000000000 ) ;
#25253=ADVANCED_FACE ( 'NONE', ( #24435 ), #42463, .F. ) ;
#25259=EDGE_CURVE ( 'NONE', #11032, #41260, #7366, .T. ) ;
#25271=EDGE_CURVE ( 'NONE', #31800, #45067, #10139, .T. ) ;
#25285=EDGE_LOOP ( 'NONE', ( #37353, #8069, #42269, #10292 ) ) ;
#25287=EDGE_CURVE ( 'NONE', #19382, #34117, #4946, .T. ) ;
#25291=DIRECTION ( 'NONE',  ( 0.000000000000000000, 0.000000000000000000, 1.000000000000000000 ) ) ;
#25292=DIRECTION ( 'NONE',  ( 0.000000000000000000, 0.7071067811865578978, 0.7071067811865372477 ) ) ;
#25329=VECTOR ( 'NONE', #4423, 999.9999999999998863 ) ;
#25341=ORIENTED_EDGE ( 'NONE', *, *, #1019, .T. ) ;
#25342=SHAPE_DEFINITION_REPRESENTATION ( #41751, #28315 ) ;
#25355=ORIENTED_EDGE ( 'NONE', *, *, #16680, .F. ) ;
#25367=CIRCLE ( 'NONE', #21676, 2.749999999999919176 ) ;
#25382=CARTESIAN_POINT ( 'NONE',  ( -338.8365100919713200, 256.5000000000001137, -197.2499999999918714 ) ) ;
#25411=CARTESIAN_POINT ( 'NONE',  ( -338.8365100919713200, 258.0940000000001078, -199.9999999999917861 ) ) ;
#25429=AXIS2_PLACEMENT_3D ( 'NONE', #29805, #30251, #19407 ) ;
#25431=VECTOR ( 'NONE', #6343, 1000.000000000000000 ) ;
#25436=CARTESIAN_POINT ( 'NONE',  ( -332.7175100919712918, 256.5000000000001137, -199.9999999999917861 ) ) ;
#25438=CIRCLE ( 'NONE', #355, 6.119000000000013095 ) ;
#25447=VERTEX_POINT ( 'NONE', #20971 ) ;
#25454=CARTESIAN_POINT ( 'NONE',  ( 441.1634899080286232, 259.9999999999999432, -199.9999999999972431 ) ) ;
#25457=ORIENTED_EDGE ( 'NONE', *, *, #16508, .T. ) ;
#25461=VERTEX_POINT ( 'NONE', #3441 ) ;
#25466=ORIENTED_EDGE ( 'NONE', *, *, #39960, .F. ) ;
#25473=EDGE_CURVE ( 'NONE', #40963, #25447, #45714, .T. ) ;
#25509=VERTEX_POINT ( 'NONE', #24665 ) ;
#25513=DIRECTION ( 'NONE',  ( 1.892425610156518354E-16, 1.000000000000000000, -0.000000000000000000 ) ) ;
#25541=CARTESIAN_POINT ( 'NONE',  ( 311.1634899080286232, 240.0000000000000000, -199.9999999999963336 ) ) ;
#25543=FACE_OUTER_BOUND ( 'NONE', #1521, .T. ) ;
#25558=CARTESIAN_POINT ( 'NONE',  ( 311.1634899080286232, 260.0000000000000000, -199.9999999999963336 ) ) ;
#25565=CARTESIAN_POINT ( 'NONE',  ( -858.8365100919713768, 256.5000000000002274, -197.2499999999882334 ) ) ;
#25575=ORIENTED_EDGE ( 'NONE', *, *, #3488, .T. ) ;
#25583=AXIS2_PLACEMENT_3D ( 'NONE', #25916, #9288, #33768 ) ;
#25599=LINE ( 'NONE', #36209, #17355 ) ;
#25600=ORIENTED_EDGE ( 'NONE', *, *, #431, .F. ) ;
#25673=DIRECTION ( 'NONE',  ( -0.000000000000000000, 1.000000000000000000, -0.000000000000000000 ) ) ;
#25749=EDGE_LOOP ( 'NONE', ( #41901, #44417, #7289, #1458 ) ) ;
#25766=CARTESIAN_POINT ( 'NONE',  ( 831.1634899080286232, 256.4999999999998863, -199.9999999999999432 ) ) ;
#25784=FACE_OUTER_BOUND ( 'NONE', #44600, .T. ) ;
#25860=ORIENTED_EDGE ( 'NONE', *, *, #2744, .F. ) ;
#25900=ORIENTED_EDGE ( 'NONE', *, *, #21009, .F. ) ;
#25911=ORIENTED_EDGE ( 'NONE', *, *, #19866, .F. ) ;
#25916=CARTESIAN_POINT ( 'NONE',  ( -338.8365100919713200, 256.5000000000001137, -199.9999999999917861 ) ) ;
#25919=VERTEX_POINT ( 'NONE', #2459 ) ;
#25937=FACE_BOUND ( 'NONE', #1929, .T. ) ;
#25975=DIRECTION ( 'NONE',  ( 0.000000000000000000, 0.000000000000000000, 1.000000000000000000 ) ) ;
#25988=CARTESIAN_POINT ( 'NONE',  ( -338.8365100919713200, 260.0000000000001137, -193.8809999999918148 ) ) ;
#26002=ORIENTED_EDGE ( 'NONE', *, *, #43103, .F. ) ;
#26017=FACE_OUTER_BOUND ( 'NONE', #10357, .T. ) ;
#26027=LINE ( 'NONE', #21667, #13050 ) ;
#26048=CARTESIAN_POINT ( 'NONE',  ( 879.9999999999992042, 259.9999999999998863, -219.9999999999999716 ) ) ;
#26055=DIRECTION ( 'NONE',  ( -0.000000000000000000, 1.000000000000000000, -0.000000000000000000 ) ) ;
#26064=EDGE_LOOP ( 'NONE', ( #29767, #35351 ) ) ;
#26079=EDGE_CURVE ( 'NONE', #10694, #40245, #7167, .T. ) ;
#26083=CYLINDRICAL_SURFACE ( 'NONE', #9105, 6.119000000000013095 ) ;
#26084=EDGE_CURVE ( 'NONE', #6776, #36186, #11586, .T. ) ;
#26093=AXIS2_PLACEMENT_3D ( 'NONE', #9794, #6783, #20637 ) ;
#26097=ADVANCED_FACE ( 'NONE', ( #8733 ), #38890, .F. ) ;
#26105=CARTESIAN_POINT ( 'NONE',  ( 311.1634899080286232, 260.0000000000000000, -208.0249999999963109 ) ) ;
#26143=ADVANCED_FACE ( 'NONE', ( #12413 ), #40594, .F. ) ;
#26181=AXIS2_PLACEMENT_3D ( 'NONE', #24980, #25673, #21983 ) ;
#26184=AXIS2_PLACEMENT_3D ( 'NONE', #5779, #19865, #10606 ) ;
#26194=ORIENTED_EDGE ( 'NONE', *, *, #11632, .F. ) ;
#26203=DIRECTION ( 'NONE',  ( 0.000000000000000000, -0.000000000000000000, -1.000000000000000000 ) ) ;
#26223=CARTESIAN_POINT ( 'NONE',  ( 311.1634899080286232, 240.0000000000000000, -202.7499999999961915 ) ) ;
#26231=DIRECTION ( 'NONE',  ( -0.000000000000000000, 1.000000000000000000, -0.000000000000000000 ) ) ;
#26239=CARTESIAN_POINT ( 'NONE',  ( 441.1634899080286232, 239.9999999999999716, -197.2499999999973852 ) ) ;
#26248=ORIENTED_EDGE ( 'NONE', *, *, #521, .T. ) ;
#26260=CONICAL_SURFACE ( 'NONE', #41663, 8.024999999999948841, 0.7853981633974337351 ) ;
#26274=VECTOR ( 'NONE', #12680, 1000.000000000000000 ) ;
#26277=ORIENTED_EDGE ( 'NONE', *, *, #24391, .T. ) ;
#26284=ORIENTED_EDGE ( 'NONE', *, *, #32600, .F. ) ;
#26291=ORIENTED_EDGE ( 'NONE', *, *, #18756, .F. ) ;
#26310=ADVANCED_FACE ( 'NONE', ( #17484 ), #20481, .F. ) ;
#26324=CARTESIAN_POINT ( 'NONE',  ( 571.1634899080285095, 258.0939999999999372, -199.9999999999981526 ) ) ;
#26331=AXIS2_PLACEMENT_3D ( 'NONE', #11388, #7698, #21327 ) ;
#26335=DIRECTION ( 'NONE',  ( -0.000000000000000000, 1.000000000000000000, -0.000000000000000000 ) ) ;
#26338=AXIS2_PLACEMENT_3D ( 'NONE', #14474, #14707, #11007 ) ;
#26360=VERTEX_POINT ( 'NONE', #10088 ) ;
#26395=AXIS2_PLACEMENT_3D ( 'NONE', #42568, #10929, #21998 ) ;
#26419=EDGE_CURVE ( 'NONE', #36186, #26697, #31563, .T. ) ;
#26430=FACE_OUTER_BOUND ( 'NONE', #6877, .T. ) ;
#26494=CYLINDRICAL_SURFACE ( 'NONE', #16745, 2.749999999999863665 ) ;
#26502=CARTESIAN_POINT ( 'NONE',  ( 701.1634899080286232, 239.9999999999999147, -199.9999999999990337 ) ) ;
#26512=DIRECTION ( 'NONE',  ( -0.000000000000000000, 1.000000000000000000, -0.000000000000000000 ) ) ;
#26518=DIRECTION ( 'NONE',  ( -0.000000000000000000, 1.000000000000000000, -0.000000000000000000 ) ) ;
#26592=PLANE ( 'NONE',  #43273 ) ;
#26602=EDGE_CURVE ( 'NONE', #22122, #30282, #28561, .T. ) ;
#26643=FACE_OUTER_BOUND ( 'NONE', #29219, .T. ) ;
#26651=DIRECTION ( 'NONE',  ( -0.000000000000000000, 1.000000000000000000, -0.000000000000000000 ) ) ;
#26655=DIRECTION ( 'NONE',  ( -0.000000000000000000, 1.000000000000000000, -0.000000000000000000 ) ) ;
#26692=ADVANCED_FACE ( 'NONE', ( #28783 ), #35696, .F. ) ;
#26697=VERTEX_POINT ( 'NONE', #29244 ) ;
#26719=ORIENTED_EDGE ( 'NONE', *, *, #431, .T. ) ;
#26735=CONICAL_SURFACE ( 'NONE', #14197, 8.024999999999948841, 0.7853981633974337351 ) ;
#26737=CARTESIAN_POINT ( 'NONE',  ( 311.1634899080286232, 240.0000000000000000, -197.2499999999964473 ) ) ;
#26778=DIRECTION ( 'NONE',  ( 0.000000000000000000, 0.000000000000000000, 1.000000000000000000 ) ) ;
#26781=DIRECTION ( 'NONE',  ( 0.000000000000000000, 0.000000000000000000, 1.000000000000000000 ) ) ;
#26817=CARTESIAN_POINT ( 'NONE',  ( -858.8365100919713768, 260.0000000000002274, -199.9999999999881481 ) ) ;
#26818=ORIENTED_EDGE ( 'NONE', *, *, #24177, .F. ) ;
#26857=ORIENTED_EDGE ( 'NONE', *, *, #28572, .F. ) ;
#26858=AXIS2_PLACEMENT_3D ( 'NONE', #23153, #34241, #6075 ) ;
#26869=CARTESIAN_POINT ( 'NONE',  ( -338.8365100919713200, 260.0000000000001137, -199.9999999999917861 ) ) ;
#26876=AXIS2_PLACEMENT_3D ( 'NONE', #11805, #33268, #1614 ) ;
#26879=CARTESIAN_POINT ( 'NONE',  ( -208.8365100919714052, 260.0000000000001137, -193.8809999999926674 ) ) ;
#26889=DIRECTION ( 'NONE',  ( -1.000000000000000000, 0.000000000000000000, 0.000000000000000000 ) ) ;
#26908=ORIENTED_EDGE ( 'NONE', *, *, #6356, .F. ) ;
#26915=VERTEX_POINT ( 'NONE', #39875 ) ;
#26916=VECTOR ( 'NONE', #29486, 1000.000000000000000 ) ;
#26922=EDGE_CURVE ( 'NONE', #3205, #13375, #31523, .T. ) ;
#26937=CIRCLE ( 'NONE', #43880, 2.749999999999919176 ) ;
#26941=AXIS2_PLACEMENT_3D ( 'NONE', #44353, #37434, #2089 ) ;
#26943=VECTOR ( 'NONE', #23004, 1000.000000000000000 ) ;
#26959=EDGE_CURVE ( 'NONE', #8042, #30282, #30129, .T. ) ;
#26973=EDGE_LOOP ( 'NONE', ( #12448, #3302, #175, #39761 ) ) ;
#26974=AXIS2_PLACEMENT_3D ( 'NONE', #14173, #17420, #28727 ) ;
#27014=VECTOR ( 'NONE', #14647, 1000.000000000000000 ) ;
#27047=CARTESIAN_POINT ( 'NONE',  ( -858.8365100919713768, 260.0000000000002274, -199.9999999999881481 ) ) ;
#27052=CIRCLE ( 'NONE', #7153, 2.749999999999919176 ) ;
#27053=ORIENTED_EDGE ( 'NONE', *, *, #3388, .T. ) ;
#27069=CARTESIAN_POINT ( 'NONE',  ( -858.8365100919713768, 260.0000000000002274, -199.9999999999881481 ) ) ;
#27112=EDGE_LOOP ( 'NONE', ( #33138, #4415, #18214, #24633 ) ) ;
#27126=VERTEX_POINT ( 'NONE', #33594 ) ;
#27186=CARTESIAN_POINT ( 'NONE',  ( -338.8365100919713200, 260.0000000000001137, -199.9999999999917861 ) ) ;
#27189=DIRECTION ( 'NONE',  ( -0.000000000000000000, 1.000000000000000000, -0.000000000000000000 ) ) ;
#27214=EDGE_LOOP ( 'NONE', ( #41155, #35305 ) ) ;
#27219=EDGE_CURVE ( 'NONE', #14468, #35726, #22639, .T. ) ;
#27224=EDGE_CURVE ( 'NONE', #3234, #7749, #12575, .T. ) ;
#27237=DIRECTION ( 'NONE',  ( -0.000000000000000000, 1.000000000000000000, -0.000000000000000000 ) ) ;
#27271=ORIENTED_EDGE ( 'NONE', *, *, #5410, .T. ) ;
#27277=CYLINDRICAL_SURFACE ( 'NONE', #36719, 2.749999999999863665 ) ;
#27295=VERTEX_POINT ( 'NONE', #37518 ) ;
#27307=CYLINDRICAL_SURFACE ( 'NONE', #17602, 6.119000000000013095 ) ;
#27409=EDGE_LOOP ( 'NONE', ( #4497, #774 ) ) ;
#27445=VECTOR ( 'NONE', #9798, 999.9999999999998863 ) ;
#27494=ADVANCED_FACE ( 'NONE', ( #35193 ), #34265, .F. ) ;
#27496=EDGE_CURVE ( 'NONE', #6776, #34351, #13495, .T. ) ;
#27505=LINE ( 'NONE', #33983, #1246 ) ;
#27522=DIRECTION ( 'NONE',  ( 0.000000000000000000, 0.000000000000000000, 1.000000000000000000 ) ) ;
#27542=VERTEX_POINT ( 'NONE', #38432 ) ;
#27552=EDGE_CURVE ( 'NONE', #20679, #18073, #32000, .T. ) ;
#27562=VERTEX_POINT ( 'NONE', #38664 ) ;
#27574=DIRECTION ( 'NONE',  ( 0.000000000000000000, 0.7071067811865578978, 0.7071067811865372477 ) ) ;
#27590=DIRECTION ( 'NONE',  ( -0.000000000000000000, 1.000000000000000000, -0.000000000000000000 ) ) ;
#27637=CARTESIAN_POINT ( 'NONE',  ( -598.8365100919716042, 260.0000000000001705, -199.9999999999899671 ) ) ;
#27642=DIRECTION ( 'NONE',  ( 0.000000000000000000, 0.000000000000000000, 1.000000000000000000 ) ) ;
#27644=ORIENTED_EDGE ( 'NONE', *, *, #20206, .F. ) ;
#27665=AXIS2_PLACEMENT_3D ( 'NONE', #5888, #13282, #41229 ) ;
#27682=ORIENTED_EDGE ( 'NONE', *, *, #11378, .F. ) ;
#27691=ADVANCED_FACE ( 'NONE', ( #41219 ), #9576, .F. ) ;
#27703=CIRCLE ( 'NONE', #26974, 6.119000000000013095 ) ;
#27740=VECTOR ( 'NONE', #42858, 1000.000000000000000 ) ;
#27745=VERTEX_POINT ( 'NONE', #17657 ) ;
#27753=AXIS2_PLACEMENT_3D ( 'NONE', #28883, #33049, #36263 ) ;
#27755=CARTESIAN_POINT ( 'NONE',  ( 51.16348990802859475, 240.0000000000000568, -199.9999999999945146 ) ) ;
#27784=ORIENTED_EDGE ( 'NONE', *, *, #26959, .T. ) ;
#27786=AXIS2_PLACEMENT_3D ( 'NONE', #5583, #4910, #5346 ) ;
#27787=ORIENTED_EDGE ( 'NONE', *, *, #34861, .T. ) ;
#27794=ORIENTED_EDGE ( 'NONE', *, *, #10834, .T. ) ;
#27800=CARTESIAN_POINT ( 'NONE',  ( 879.9999999999992042, 259.9999999999998863, -219.9999999999999716 ) ) ;
#27812=DIRECTION ( 'NONE',  ( -0.000000000000000000, 1.000000000000000000, -0.000000000000000000 ) ) ;
#27829=VECTOR ( 'NONE', #26651, 1000.000000000000000 ) ;
#27863=CYLINDRICAL_SURFACE ( 'NONE', #22523, 6.119000000000013095 ) ;
#27885=CARTESIAN_POINT ( 'NONE',  ( 831.1634899080286232, 259.9999999999998863, -199.9999999999999432 ) ) ;
#27919=DIRECTION ( 'NONE',  ( 1.000000000000000000, 0.000000000000000000, 0.000000000000000000 ) ) ;
#27947=CIRCLE ( 'NONE', #33847, 8.024999999999948841 ) ;
#27953=DIRECTION ( 'NONE',  ( -0.000000000000000000, 1.000000000000000000, -0.000000000000000000 ) ) ;
#27971=DIRECTION ( 'NONE',  ( 0.000000000000000000, 0.000000000000000000, 1.000000000000000000 ) ) ;
#27999=ORIENTED_EDGE ( 'NONE', *, *, #18226, .T. ) ;
#28025=LINE ( 'NONE', #41216, #43994 ) ;
#28032=CARTESIAN_POINT ( 'NONE',  ( 311.1634899080286232, 258.0939999999999941, -193.8809999999963338 ) ) ;
#28035=EDGE_CURVE ( 'NONE', #29766, #34711, #10712, .T. ) ;
#28074=CARTESIAN_POINT ( 'NONE',  ( -598.8365100919716042, 256.5000000000001705, -199.9999999999899671 ) ) ;
#28078=EDGE_LOOP ( 'NONE', ( #39680, #38581 ) ) ;
#28109=EDGE_CURVE ( 'NONE', #33219, #17388, #32744, .T. ) ;
#28121=DIRECTION ( 'NONE',  ( -0.000000000000000000, 1.000000000000000000, -0.000000000000000000 ) ) ;
#28143=EDGE_CURVE ( 'NONE', #35726, #33524, #43704, .T. ) ;
#28152=DIRECTION ( 'NONE',  ( 0.000000000000000000, 0.000000000000000000, 1.000000000000000000 ) ) ;
#28187=DIRECTION ( 'NONE',  ( -0.000000000000000000, 1.000000000000000000, -0.000000000000000000 ) ) ;
#28189=LINE ( 'NONE', #17811, #13057 ) ;
#28210=FACE_OUTER_BOUND ( 'NONE', #32215, .T. ) ;
#28258=DIRECTION ( 'NONE',  ( 0.000000000000000000, 0.000000000000000000, 1.000000000000000000 ) ) ;
#28279=VERTEX_POINT ( 'NONE', #5589 ) ;
#28297=VERTEX_POINT ( 'NONE', #12524 ) ;
#28314=CARTESIAN_POINT ( 'NONE',  ( -728.8365100919714905, 258.0940000000001646, -193.8809999999890863 ) ) ;
#28315=SHAPE_REPRESENTATION ( 'Lower Fixed Bed Shear Blade', ( #26858 ), #32791 ) ;
#28320=LINE ( 'NONE', #42661, #41070 ) ;
#28374=AXIS2_PLACEMENT_3D ( 'NONE', #43826, #26512, #12886 ) ;
#28380=CYLINDRICAL_SURFACE ( 'NONE', #21773, 2.749999999999863665 ) ;
#28405=AXIS2_PLACEMENT_3D ( 'NONE', #16628, #38736, #34152 ) ;
#28426=ORIENTED_EDGE ( 'NONE', *, *, #32534, .T. ) ;
#28444=AXIS2_PLACEMENT_3D ( 'NONE', #17617, #43177, #36025 ) ;
#28468=ORIENTED_EDGE ( 'NONE', *, *, #8094, .T. ) ;
#28470=CONICAL_SURFACE ( 'NONE', #14473, 8.025000000000003908, 0.7853981633974482790 ) ;
#28485=DIRECTION ( 'NONE',  ( -0.000000000000000000, 1.000000000000000000, -0.000000000000000000 ) ) ;
#28486=VECTOR ( 'NONE', #16151, 1000.000000000000000 ) ;
#28490=FACE_OUTER_BOUND ( 'NONE', #19253, .T. ) ;
#28518=CARTESIAN_POINT ( 'NONE',  ( 701.1634899080286232, 259.9999999999999432, -191.9749999999990848 ) ) ;
#28545=DIRECTION ( 'NONE',  ( -0.000000000000000000, 1.000000000000000000, -0.000000000000000000 ) ) ;
#28553=AXIS2_PLACEMENT_3D ( 'NONE', #27069, #45080, #13658 ) ;
#28554=DIRECTION ( 'NONE',  ( 0.000000000000000000, 0.000000000000000000, 1.000000000000000000 ) ) ;
#28555=DIRECTION ( 'NONE',  ( 0.000000000000000000, 0.000000000000000000, 1.000000000000000000 ) ) ;
#28560=FACE_BOUND ( 'NONE', #35800, .T. ) ;
#28561=CIRCLE ( 'NONE', #3500, 2.749999999999919176 ) ;
#28572=EDGE_CURVE ( 'NONE', #42341, #2204, #3290, .T. ) ;
#28578=VECTOR ( 'NONE', #18915, 1000.000000000000000 ) ;
#28622=VECTOR ( 'NONE', #7458, 1000.000000000000000 ) ;
#28623=CARTESIAN_POINT ( 'NONE',  ( -858.8365100919713768, 260.0000000000002274, -199.9999999999881481 ) ) ;
#28628=EDGE_CURVE ( 'NONE', #7001, #40012, #16360, .T. ) ;
#28653=VECTOR ( 'NONE', #34349, 1000.000000000000000 ) ;
#28668=ORIENTED_EDGE ( 'NONE', *, *, #23757, .T. ) ;
#28680=FACE_OUTER_BOUND ( 'NONE', #31430, .T. ) ;
#28696=ADVANCED_FACE ( 'NONE', ( #37606, #2040 ), #43842, .F. ) ;
#28698=ORIENTED_EDGE ( 'NONE', *, *, #38814, .T. ) ;
#28723=LINE ( 'NONE', #11162, #30711 ) ;
#28727=DIRECTION ( 'NONE',  ( 0.000000000000000000, 0.000000000000000000, 1.000000000000000000 ) ) ;
#28728=CARTESIAN_POINT ( 'NONE',  ( -78.83651009197140525, 258.0940000000000509, -193.8809999999935769 ) ) ;
#28737=DIRECTION ( 'NONE',  ( 1.892425610156518354E-16, 1.000000000000000000, -0.000000000000000000 ) ) ;
#28759=CARTESIAN_POINT ( 'NONE',  ( 831.1634899080286232, 239.9999999999998863, -199.9999999999999432 ) ) ;
#28761=EDGE_LOOP ( 'NONE', ( #668, #18993 ) ) ;
#28783=FACE_OUTER_BOUND ( 'NONE', #13467, .T. ) ;
#28784=CARTESIAN_POINT ( 'NONE',  ( -208.8365100919714052, 256.5000000000001137, -197.2499999999927809 ) ) ;
#28786=FACE_OUTER_BOUND ( 'NONE', #8435, .T. ) ;
#28789=DIRECTION ( 'NONE',  ( 0.000000000000000000, -1.000000000000000000, 0.000000000000000000 ) ) ;
#28838=PLANE ( 'NONE',  #20082 ) ;
#28845=DIRECTION ( 'NONE',  ( 0.000000000000000000, -1.000000000000000000, 0.000000000000000000 ) ) ;
#28871=ORIENTED_EDGE ( 'NONE', *, *, #29650, .F. ) ;
#28883=CARTESIAN_POINT ( 'NONE',  ( 51.16348990802859475, 258.0940000000000509, -199.9999999999945146 ) ) ;
#28910=FACE_OUTER_BOUND ( 'NONE', #7233, .T. ) ;
#28917=FACE_OUTER_BOUND ( 'NONE', #8158, .T. ) ;
#28933=EDGE_CURVE ( 'NONE', #10119, #13600, #23726, .T. ) ;
#28937=VERTEX_POINT ( 'NONE', #41999 ) ;
#28948=VERTEX_POINT ( 'NONE', #38077 ) ;
#28955=EDGE_CURVE ( 'NONE', #9099, #30459, #30544, .T. ) ;
#28972=EDGE_CURVE ( 'NONE', #9876, #16943, #1047, .T. ) ;
#28976=EDGE_CURVE ( 'NONE', #44542, #16836, #20515, .T. ) ;
#28986=ORIENTED_EDGE ( 'NONE', *, *, #13710, .T. ) ;
#29003=LINE ( 'NONE', #43318, #27740 ) ;
#29004=AXIS2_PLACEMENT_3D ( 'NONE', #36387, #4749, #15388 ) ;
#29032=VERTEX_POINT ( 'NONE', #11302 ) ;
#29034=CIRCLE ( 'NONE', #37121, 2.749999999999808153 ) ;
#29065=DIRECTION ( 'NONE',  ( 0.000000000000000000, 0.000000000000000000, 1.000000000000000000 ) ) ;
#29131=CARTESIAN_POINT ( 'NONE',  ( 701.1634899080286232, 259.9999999999999432, -199.9999999999990337 ) ) ;
#29138=ADVANCED_FACE ( 'NONE', ( #25144 ), #36458, .F. ) ;
#29179=AXIS2_PLACEMENT_3D ( 'NONE', #33060, #43876, #39986 ) ;
#29219=EDGE_LOOP ( 'NONE', ( #252, #19722 ) ) ;
#29244=CARTESIAN_POINT ( 'NONE',  ( 571.1634899080285095, 258.0939999999999372, -193.8809999999981528 ) ) ;
#29251=FACE_BOUND ( 'NONE', #9616, .T. ) ;
#29254=EDGE_CURVE ( 'NONE', #30100, #9272, #323, .T. ) ;
#29256=CARTESIAN_POINT ( 'NONE',  ( 311.1634899080286232, 260.0000000000000000, -199.9999999999963336 ) ) ;
#29270=DIRECTION ( 'NONE',  ( 0.000000000000000000, 0.000000000000000000, 1.000000000000000000 ) ) ;
#29288=CIRCLE ( 'NONE', #27786, 8.025000000000003908 ) ;
#29341=EDGE_LOOP ( 'NONE', ( #32895, #7570, #16650, #34982 ) ) ;
#29342=VERTEX_POINT ( 'NONE', #15238 ) ;
#29353=CARTESIAN_POINT ( 'NONE',  ( -728.8365100919714905, 260.0000000000001705, -199.9999999999890861 ) ) ;
#29360=EDGE_CURVE ( 'NONE', #10119, #40963, #4823, .T. ) ;
#29383=AXIS2_PLACEMENT_3D ( 'NONE', #27885, #6413, #45204 ) ;
#29392=EDGE_LOOP ( 'NONE', ( #36406, #39224, #1102, #2489 ) ) ;
#29413=CARTESIAN_POINT ( 'NONE',  ( -858.8365100919713768, 260.0000000000002274, -208.0249999999880970 ) ) ;
#29419=DIRECTION ( 'NONE',  ( -0.000000000000000000, 1.000000000000000000, -0.000000000000000000 ) ) ;
#29441=AXIS2_PLACEMENT_3D ( 'NONE', #37877, #12701, #26781 ) ;
#29443=ORIENTED_EDGE ( 'NONE', *, *, #34861, .F. ) ;
#29462=CARTESIAN_POINT ( 'NONE',  ( 311.1634899080286232, 256.5000000000000000, -197.2499999999963904 ) ) ;
#29486=DIRECTION ( 'NONE',  ( 8.659560562354869996E-17, 0.7071067811865526798, -0.7071067811865423547 ) ) ;
#29549=ADVANCED_FACE ( 'NONE', ( #44528 ), #18798, .F. ) ;
#29556=ORIENTED_EDGE ( 'NONE', *, *, #569, .T. ) ;
#29581=CARTESIAN_POINT ( 'NONE',  ( 51.16348990802859475, 260.0000000000000568, -199.9999999999945146 ) ) ;
#29587=DIRECTION ( 'NONE',  ( -0.000000000000000000, 1.000000000000000000, -0.000000000000000000 ) ) ;
#29596=CYLINDRICAL_SURFACE ( 'NONE', #35051, 2.749999999999863665 ) ;
#29605=ORIENTED_EDGE ( 'NONE', *, *, #5829, .T. ) ;
#29650=EDGE_CURVE ( 'NONE', #9272, #8247, #44297, .T. ) ;
#29659=ORIENTED_EDGE ( 'NONE', *, *, #28628, .F. ) ;
#29673=DIRECTION ( 'NONE',  ( -0.000000000000000000, 1.000000000000000000, -0.000000000000000000 ) ) ;
#29711=VECTOR ( 'NONE', #44447, 999.9999999999998863 ) ;
#29741=AXIS2_PLACEMENT_3D ( 'NONE', #724, #35824, #24103 ) ;
#29755=CARTESIAN_POINT ( 'NONE',  ( -338.8365100919713200, 260.0000000000001137, -199.9999999999917861 ) ) ;
#29759=VERTEX_POINT ( 'NONE', #24405 ) ;
#29765=EDGE_CURVE ( 'NONE', #21723, #40483, #4058, .T. ) ;
#29766=VERTEX_POINT ( 'NONE', #23945 ) ;
#29767=ORIENTED_EDGE ( 'NONE', *, *, #21597, .F. ) ;
#29805=CARTESIAN_POINT ( 'NONE',  ( 51.16348990802859475, 256.5000000000000568, -199.9999999999945146 ) ) ;
#29806=FACE_OUTER_BOUND ( 'NONE', #13200, .T. ) ;
#29809=EDGE_CURVE ( 'NONE', #41260, #42341, #6859, .T. ) ;
#29815=CARTESIAN_POINT ( 'NONE',  ( -338.8365100919713200, 260.0000000000001137, -199.9999999999917861 ) ) ;
#29856=VECTOR ( 'NONE', #19859, 1000.000000000000114 ) ;
#29863=FACE_OUTER_BOUND ( 'NONE', #41667, .T. ) ;
#29872=EDGE_LOOP ( 'NONE', ( #34257, #19720 ) ) ;
#29892=CYLINDRICAL_SURFACE ( 'NONE', #45445, 2.749999999999863665 ) ;
#29898=ORIENTED_EDGE ( 'NONE', *, *, #2930, .F. ) ;
#29904=DIRECTION ( 'NONE',  ( -0.000000000000000000, 1.000000000000000000, -0.000000000000000000 ) ) ;
#29907=FACE_BOUND ( 'NONE', #12521, .T. ) ;
#29922=CARTESIAN_POINT ( 'NONE',  ( 441.1634899080286232, 259.9999999999999432, -193.8809999999972433 ) ) ;
#29936=CARTESIAN_POINT ( 'NONE',  ( 181.1634899080285948, 256.5000000000000000, -193.8809999999953959 ) ) ;
#29960=DIRECTION ( 'NONE',  ( 0.000000000000000000, 0.000000000000000000, 1.000000000000000000 ) ) ;
#29996=VERTEX_POINT ( 'NONE', #14259 ) ;
#30005=ORIENTED_EDGE ( 'NONE', *, *, #19848, .T. ) ;
#30008=ORIENTED_EDGE ( 'NONE', *, *, #4128, .T. ) ;
#30010=CARTESIAN_POINT ( 'NONE',  ( -858.8365100919713768, 260.0000000000002274, -193.8809999999881768 ) ) ;
#30012=VECTOR ( 'NONE', #10361, 1000.000000000000000 ) ;
#30013=DIRECTION ( 'NONE',  ( 0.000000000000000000, 0.000000000000000000, 1.000000000000000000 ) ) ;
#30057=ORIENTED_EDGE ( 'NONE', *, *, #6661, .T. ) ;
#30073=DIRECTION ( 'NONE',  ( 0.000000000000000000, 0.000000000000000000, 1.000000000000000000 ) ) ;
#30075=DIRECTION ( 'NONE',  ( -0.000000000000000000, 1.000000000000000000, -0.000000000000000000 ) ) ;
#30076=ORIENTED_EDGE ( 'NONE', *, *, #14334, .F. ) ;
#30087=AXIS2_PLACEMENT_3D ( 'NONE', #20615, #34710, #3068 ) ;
#30100=VERTEX_POINT ( 'NONE', #39210 ) ;
#30113=ADVANCED_FACE ( 'NONE', ( #25784 ), #13647, .F. ) ;
#30117=CIRCLE ( 'NONE', #20558, 8.024999999999948841 ) ;
#30129=LINE ( 'NONE', #19275, #27829 ) ;
#30134=DIRECTION ( 'NONE',  ( -0.000000000000000000, 1.000000000000000000, -0.000000000000000000 ) ) ;
#30161=FACE_BOUND ( 'NONE', #32918, .T. ) ;
#30177=CARTESIAN_POINT ( 'NONE',  ( 51.16348990802859475, 260.0000000000000568, -199.9999999999945146 ) ) ;
#30199=DIRECTION ( 'NONE',  ( -0.000000000000000000, 1.000000000000000000, -0.000000000000000000 ) ) ;
#30214=AXIS2_PLACEMENT_3D ( 'NONE', #26869, #6775, #34949 ) ;
#30245=LINE ( 'NONE', #40439, #4096 ) ;
#30251=DIRECTION ( 'NONE',  ( -0.000000000000000000, 1.000000000000000000, -0.000000000000000000 ) ) ;
#30266=ADVANCED_FACE ( 'NONE', ( #38989 ), #21415, .F. ) ;
#30269=DIRECTION ( 'NONE',  ( 1.892425610156518354E-16, 1.000000000000000000, -0.000000000000000000 ) ) ;
#30282=VERTEX_POINT ( 'NONE', #25565 ) ;
#30287=LINE ( 'NONE', #22900, #38148 ) ;
#30290=EDGE_LOOP ( 'NONE', ( #40686, #17638 ) ) ;
#30296=DIRECTION ( 'NONE',  ( -0.000000000000000000, 1.000000000000000000, -0.000000000000000000 ) ) ;
#30338=DIRECTION ( 'NONE',  ( 0.000000000000000000, 0.000000000000000000, 1.000000000000000000 ) ) ;
#30340=FACE_OUTER_BOUND ( 'NONE', #8519, .T. ) ;
#30352=DIRECTION ( 'NONE',  ( 0.000000000000000000, 0.000000000000000000, 1.000000000000000000 ) ) ;
#30393=ORIENTED_EDGE ( 'NONE', *, *, #16443, .F. ) ;
#30432=VECTOR ( 'NONE', #36216, 1000.000000000000000 ) ;
#30452=ORIENTED_EDGE ( 'NONE', *, *, #4052, .T. ) ;
#30459=VERTEX_POINT ( 'NONE', #16295 ) ;
#30468=DIRECTION ( 'NONE',  ( 0.000000000000000000, 0.000000000000000000, 1.000000000000000000 ) ) ;
#30496=DIRECTION ( 'NONE',  ( 0.000000000000000000, 0.000000000000000000, 1.000000000000000000 ) ) ;
#30514=CARTESIAN_POINT ( 'NONE',  ( 831.1634899080286232, 256.4999999999998863, -206.1189999999999429 ) ) ;
#30515=FACE_OUTER_BOUND ( 'NONE', #40153, .T. ) ;
#30533=FACE_OUTER_BOUND ( 'NONE', #25749, .T. ) ;
#30544=CIRCLE ( 'NONE', #20949, 8.025000000000003908 ) ;
#30554=VERTEX_POINT ( 'NONE', #26239 ) ;
#30559=ORIENTED_EDGE ( 'NONE', *, *, #2117, .F. ) ;
#30575=DIRECTION ( 'NONE',  ( -1.000000000000000000, 0.000000000000000000, -0.000000000000000000 ) ) ;
#30580=DIRECTION ( 'NONE',  ( 1.892425610156518354E-16, 1.000000000000000000, -0.000000000000000000 ) ) ;
#30589=AXIS2_PLACEMENT_3D ( 'NONE', #36123, #1006, #44468 ) ;
#30604=AXIS2_PLACEMENT_3D ( 'NONE', #5311, #29587, #43663 ) ;
#30638=DIRECTION ( 'NONE',  ( -0.000000000000000000, 1.000000000000000000, -0.000000000000000000 ) ) ;
#30641=EDGE_CURVE ( 'NONE', #24881, #12460, #8466, .T. ) ;
#30655=ORIENTED_EDGE ( 'NONE', *, *, #24599, .F. ) ;
#30674=ORIENTED_EDGE ( 'NONE', *, *, #13409, .F. ) ;
#30680=VERTEX_POINT ( 'NONE', #20884 ) ;
#30689=CONICAL_SURFACE ( 'NONE', #24039, 8.025000000000003908, 0.7853981633974482790 ) ;
#30690=ADVANCED_FACE ( 'NONE', ( #41931, #6583 ), #2894, .F. ) ;
#30711=VECTOR ( 'NONE', #25234, 1000.000000000000000 ) ;
#30723=CARTESIAN_POINT ( 'NONE',  ( -338.8365100919713200, 258.0940000000001078, -199.9999999999917861 ) ) ;
#30742=FACE_OUTER_BOUND ( 'NONE', #16134, .T. ) ;
#30743=ORIENTED_EDGE ( 'NONE', *, *, #38265, .F. ) ;
#30764=CARTESIAN_POINT ( 'NONE',  ( -879.9999999999992042, 260.0000000000002274, -179.9999999999999716 ) ) ;
#30765=ORIENTED_EDGE ( 'NONE', *, *, #1009, .T. ) ;
#30769=CARTESIAN_POINT ( 'NONE',  ( 831.1634899080286232, 259.9999999999998863, -199.9999999999999432 ) ) ;
#30775=AXIS2_PLACEMENT_3D ( 'NONE', #23186, #40996, #11757 ) ;
#30790=VERTEX_POINT ( 'NONE', #41243 ) ;
#30815=DIRECTION ( 'NONE',  ( -0.000000000000000000, 1.000000000000000000, -0.000000000000000000 ) ) ;
#30819=DIRECTION ( 'NONE',  ( 0.000000000000000000, 0.000000000000000000, 1.000000000000000000 ) ) ;
#30823=DIRECTION ( 'NONE',  ( -0.000000000000000000, 1.000000000000000000, -0.000000000000000000 ) ) ;
#30853=EDGE_LOOP ( 'NONE', ( #12685, #32425, #32802, #10687 ) ) ;
#30902=ORIENTED_EDGE ( 'NONE', *, *, #27224, .T. ) ;
#30903=EDGE_CURVE ( 'NONE', #9887, #11032, #12917, .T. ) ;
#30908=ORIENTED_EDGE ( 'NONE', *, *, #28035, .T. ) ;
#30929=DIRECTION ( 'NONE',  ( -0.000000000000000000, 1.000000000000000000, -0.000000000000000000 ) ) ;
#30933=CARTESIAN_POINT ( 'NONE',  ( 311.1634899080286232, 258.0939999999999941, -199.9999999999963336 ) ) ;
#30986=ORIENTED_EDGE ( 'NONE', *, *, #9750, .F. ) ;
#31002=FACE_BOUND ( 'NONE', #15580, .T. ) ;
#31025=ORIENTED_EDGE ( 'NONE', *, *, #34881, .F. ) ;
#31042=CARTESIAN_POINT ( 'NONE',  ( 181.1634899080285948, 260.0000000000000000, -206.1189999999954239 ) ) ;
#31056=DIRECTION ( 'NONE',  ( 0.000000000000000000, -0.000000000000000000, -1.000000000000000000 ) ) ;
#31065=ORIENTED_EDGE ( 'NONE', *, *, #43267, .F. ) ;
#31071=VERTEX_POINT ( 'NONE', #10737 ) ;
#31104=EDGE_CURVE ( 'NONE', #8149, #31071, #42426, .T. ) ;
#31105=DIRECTION ( 'NONE',  ( 1.892425610156518354E-16, 1.000000000000000000, -0.000000000000000000 ) ) ;
#31106=FACE_OUTER_BOUND ( 'NONE', #14096, .T. ) ;
#31142=ORIENTED_EDGE ( 'NONE', *, *, #9484, .T. ) ;
#31144=DIRECTION ( 'NONE',  ( 1.000000000000000000, -1.880165489482579047E-16, 0.000000000000000000 ) ) ;
#31148=EDGE_CURVE ( 'NONE', #6808, #22371, #38021, .T. ) ;
#31151=ORIENTED_EDGE ( 'NONE', *, *, #24693, .T. ) ;
#31198=CIRCLE ( 'NONE', #9802, 6.118999999999985562 ) ;
#31200=ORIENTED_EDGE ( 'NONE', *, *, #29809, .T. ) ;
#31226=FACE_BOUND ( 'NONE', #28761, .T. ) ;
#31263=DIRECTION ( 'NONE',  ( 0.000000000000000000, 0.000000000000000000, 1.000000000000000000 ) ) ;
#31266=AXIS2_PLACEMENT_3D ( 'NONE', #2650, #37529, #16512 ) ;
#31268=CARTESIAN_POINT ( 'NONE',  ( 571.1634899080285095, 259.9999999999999432, -206.1189999999981239 ) ) ;
#31275=CARTESIAN_POINT ( 'NONE',  ( 51.16348990802859475, 260.0000000000000568, -193.8809999999945148 ) ) ;
#31299=EDGE_LOOP ( 'NONE', ( #4338, #23106, #31151, #2109 ) ) ;
#31310=AXIS2_PLACEMENT_3D ( 'NONE', #12446, #1584, #36925 ) ;
#31317=VECTOR ( 'NONE', #1967, 1000.000000000000000 ) ;
#31328=CARTESIAN_POINT ( 'NONE',  ( 51.16348990802859475, 256.5000000000000568, -202.7499999999944009 ) ) ;
#31353=DIRECTION ( 'NONE',  ( -0.000000000000000000, 1.000000000000000000, -0.000000000000000000 ) ) ;
#31360=DIRECTION ( 'NONE',  ( -0.000000000000000000, 1.000000000000000000, -0.000000000000000000 ) ) ;
#31374=AXIS2_PLACEMENT_3D ( 'NONE', #37415, #26335, #16389 ) ;
#31376=ORIENTED_EDGE ( 'NONE', *, *, #43267, .T. ) ;
#31379=CYLINDRICAL_SURFACE ( 'NONE', #24819, 2.749999999999835687 ) ;
#31381=CARTESIAN_POINT ( 'NONE',  ( -338.8365100919713200, 256.5000000000001137, -206.1189999999917859 ) ) ;
#31397=AXIS2_PLACEMENT_3D ( 'NONE', #1218, #39593, #7702 ) ;
#31419=CARTESIAN_POINT ( 'NONE',  ( 311.1634899080286232, 260.0000000000000000, -199.9999999999963336 ) ) ;
#31430=EDGE_LOOP ( 'NONE', ( #43462, #37841, #31142, #32780 ) ) ;
#31441=EDGE_CURVE ( 'NONE', #8149, #30790, #39619, .T. ) ;
#31446=EDGE_CURVE ( 'NONE', #5298, #10119, #40050, .T. ) ;
#31450=ADVANCED_FACE ( 'NONE', ( #9313 ), #15563, .F. ) ;
#31460=FACE_BOUND ( 'NONE', #17404, .T. ) ;
#31466=AXIS2_PLACEMENT_3D ( 'NONE', #23114, #8832, #4909 ) ;
#31473=CIRCLE ( 'NONE', #20384, 2.749999999999891642 ) ;
#31488=ORIENTED_EDGE ( 'NONE', *, *, #8063, .F. ) ;
#31518=VECTOR ( 'NONE', #9082, 1000.000000000000000 ) ;
#31523=CIRCLE ( 'NONE', #26338, 2.749999999999919176 ) ;
#31558=ORIENTED_EDGE ( 'NONE', *, *, #20111, .T. ) ;
#31563=LINE ( 'NONE', #20692, #32216 ) ;
#31576=DIRECTION ( 'NONE',  ( 0.000000000000000000, 0.000000000000000000, 1.000000000000000000 ) ) ;
#31592=ORIENTED_EDGE ( 'NONE', *, *, #42741, .T. ) ;
#31617=EDGE_LOOP ( 'NONE', ( #41768, #27999, #14986, #35446 ) ) ;
#31621=DIRECTION ( 'NONE',  ( -0.000000000000000000, 1.000000000000000000, -0.000000000000000000 ) ) ;
#31629=CARTESIAN_POINT ( 'NONE',  ( 701.1634899080286232, 256.4999999999999432, -197.2499999999991189 ) ) ;
#31638=ORIENTED_EDGE ( 'NONE', *, *, #35350, .T. ) ;
#31666=DIRECTION ( 'NONE',  ( -0.000000000000000000, 1.000000000000000000, -0.000000000000000000 ) ) ;
#31678=FACE_BOUND ( 'NONE', #9946, .T. ) ;
#31696=FACE_OUTER_BOUND ( 'NONE', #19096, .T. ) ;
#31697=ORIENTED_EDGE ( 'NONE', *, *, #27219, .F. ) ;
#31715=ORIENTED_EDGE ( 'NONE', *, *, #34881, .T. ) ;
#31740=CARTESIAN_POINT ( 'NONE',  ( 701.1634899080286232, 259.9999999999999432, -199.9999999999990337 ) ) ;
#31750=ORIENTED_EDGE ( 'NONE', *, *, #34286, .T. ) ;
#31791=CARTESIAN_POINT ( 'NONE',  ( -858.8365100919713768, 258.0940000000002215, -199.9999999999881481 ) ) ;
#31800=VERTEX_POINT ( 'NONE', #33560 ) ;
#31864=ORIENTED_EDGE ( 'NONE', *, *, #1019, .F. ) ;
#31873=ORIENTED_EDGE ( 'NONE', *, *, #18116, .F. ) ;
#31895=CARTESIAN_POINT ( 'NONE',  ( -78.83651009197140525, 258.0940000000000509, -199.9999999999936051 ) ) ;
#31910=ORIENTED_EDGE ( 'NONE', *, *, #4150, .T. ) ;
#31915=VECTOR ( 'NONE', #16966, 1000.000000000000000 ) ;
#31944=CARTESIAN_POINT ( 'NONE',  ( 441.1634899080286232, 256.4999999999999432, -202.7499999999971578 ) ) ;
#31947=CONICAL_SURFACE ( 'NONE', #29741, 8.024999999999948841, 0.7853981633974337351 ) ;
#31948=CARTESIAN_POINT ( 'NONE',  ( 571.1634899080285095, 256.4999999999999432, -206.1189999999981239 ) ) ;
#31984=CONICAL_SURFACE ( 'NONE', #1737, 8.025000000000003908, 0.7853981633974482790 ) ;
#31987=CIRCLE ( 'NONE', #18623, 6.118999999999985562 ) ;
#31997=DIRECTION ( 'NONE',  ( -0.000000000000000000, 1.000000000000000000, -0.000000000000000000 ) ) ;
#32000=CIRCLE ( 'NONE', #38642, 2.749999999999863665 ) ;
#32004=DIRECTION ( 'NONE',  ( -0.000000000000000000, 1.000000000000000000, -0.000000000000000000 ) ) ;
#32019=CARTESIAN_POINT ( 'NONE',  ( 311.1634899080286232, 240.0000000000000000, -199.9999999999963336 ) ) ;
#32029=ORIENTED_EDGE ( 'NONE', *, *, #18681, .T. ) ;
#32034=ORIENTED_EDGE ( 'NONE', *, *, #8094, .F. ) ;
#32036=ADVANCED_FACE ( 'NONE', ( #22362 ), #1575, .F. ) ;
#32038=AXIS2_PLACEMENT_3D ( 'NONE', #32019, #14252, #35484 ) ;
#32058=VECTOR ( 'NONE', #43489, 1000.000000000000000 ) ;
#32070=PLANE ( 'NONE',  #19690 ) ;
#32075=CIRCLE ( 'NONE', #7028, 6.118999999999985562 ) ;
#32078=DIRECTION ( 'NONE',  ( -1.000000000000000000, 0.000000000000000000, 0.000000000000000000 ) ) ;
#32096=ORIENTED_EDGE ( 'NONE', *, *, #20154, .F. ) ;
#32101=CONICAL_SURFACE ( 'NONE', #29179, 8.024999999999948841, 0.7853981633974337351 ) ;
#32108=ADVANCED_FACE ( 'NONE', ( #22151 ), #15675, .F. ) ;
#32109=AXIS2_PLACEMENT_3D ( 'NONE', #40716, #37245, #36583 ) ;
#32115=ORIENTED_EDGE ( 'NONE', *, *, #24682, .T. ) ;
#32120=FACE_OUTER_BOUND ( 'NONE', #9089, .T. ) ;
#32129=AXIS2_PLACEMENT_3D ( 'NONE', #17922, #11221, #3833 ) ;
#32136=LINE ( 'NONE', #7656, #33572 ) ;
#32145=CIRCLE ( 'NONE', #6325, 6.118999999999985562 ) ;
#32161=CYLINDRICAL_SURFACE ( 'NONE', #24913, 6.118999999999985562 ) ;
#32165=CIRCLE ( 'NONE', #14364, 2.749999999999919176 ) ;
#32215=EDGE_LOOP ( 'NONE', ( #2496, #9234, #1572, #19898 ) ) ;
#32216=VECTOR ( 'NONE', #16797, 1000.000000000000000 ) ;
#32230=ORIENTED_EDGE ( 'NONE', *, *, #27552, .T. ) ;
#32246=CONICAL_SURFACE ( 'NONE', #18250, 8.025000000000003908, 0.7853981633974410625 ) ;
#32253=CARTESIAN_POINT ( 'NONE',  ( -858.8365100919713768, 256.5000000000002274, -199.9999999999881481 ) ) ;
#32266=CARTESIAN_POINT ( 'NONE',  ( -858.8365100919713768, 240.0000000000002274, -202.7499999999880345 ) ) ;
#32274=ORIENTED_EDGE ( 'NONE', *, *, #29765, .T. ) ;
#32286=EDGE_LOOP ( 'NONE', ( #21158, #21079 ) ) ;
#32288=ORIENTED_EDGE ( 'NONE', *, *, #14771, .F. ) ;
#32290=ADVANCED_FACE ( 'NONE', ( #42311 ), #30689, .F. ) ;
#32308=DIRECTION ( 'NONE',  ( 0.000000000000000000, 0.000000000000000000, 1.000000000000000000 ) ) ;
#32321=ADVANCED_FACE ( 'NONE', ( #15468 ), #35154, .F. ) ;
#32338=ORIENTED_EDGE ( 'NONE', *, *, #2117, .T. ) ;
#32357=CARTESIAN_POINT ( 'NONE',  ( -858.8365100919713768, 256.5000000000002274, -199.9999999999881481 ) ) ;
#32371=EDGE_CURVE ( 'NONE', #27126, #15586, #20358, .T. ) ;
#32380=CYLINDRICAL_SURFACE ( 'NONE', #23895, 6.118999999999985562 ) ;
#32411=VERTEX_POINT ( 'NONE', #26737 ) ;
#32415=ORIENTED_EDGE ( 'NONE', *, *, #29809, .F. ) ;
#32420=DIRECTION ( 'NONE',  ( -1.880165489482579047E-16, -1.000000000000000000, -0.000000000000000000 ) ) ;
#32423=DIRECTION ( 'NONE',  ( -0.000000000000000000, 1.000000000000000000, -0.000000000000000000 ) ) ;
#32425=ORIENTED_EDGE ( 'NONE', *, *, #20172, .T. ) ;
#32469=DIRECTION ( 'NONE',  ( 8.659560562354807133E-17, 0.7071067811865578978, -0.7071067811865372477 ) ) ;
#32479=DIRECTION ( 'NONE',  ( -0.000000000000000000, 1.000000000000000000, -0.000000000000000000 ) ) ;
#32511=VERTEX_POINT ( 'NONE', #1792 ) ;
#32530=DIRECTION ( 'NONE',  ( -0.000000000000000000, 1.000000000000000000, -0.000000000000000000 ) ) ;
#32534=EDGE_CURVE ( 'NONE', #33435, #35726, #2032, .T. ) ;
#32540=CYLINDRICAL_SURFACE ( 'NONE', #7182, 2.749999999999863665 ) ;
#32545=DIRECTION ( 'NONE',  ( -0.000000000000000000, 1.000000000000000000, -0.000000000000000000 ) ) ;
#32552=DIRECTION ( 'NONE',  ( 0.000000000000000000, 0.000000000000000000, 1.000000000000000000 ) ) ;
#32560=ORIENTED_EDGE ( 'NONE', *, *, #35350, .F. ) ;
#32582=CYLINDRICAL_SURFACE ( 'NONE', #41810, 2.749999999999863665 ) ;
#32600=EDGE_CURVE ( 'NONE', #16943, #9876, #18902, .T. ) ;
#32616=EDGE_LOOP ( 'NONE', ( #3978, #12962, #18610, #32274 ) ) ;
#32639=LINE ( 'NONE', #4249, #14511 ) ;
#32643=CYLINDRICAL_SURFACE ( 'NONE', #31397, 2.749999999999863665 ) ;
#32654=CARTESIAN_POINT ( 'NONE',  ( -338.8365100919713200, 260.0000000000001137, -202.7499999999916724 ) ) ;
#32679=ORIENTED_EDGE ( 'NONE', *, *, #20172, .F. ) ;
#32688=VERTEX_POINT ( 'NONE', #24192 ) ;
#32698=CIRCLE ( 'NONE', #13505, 2.749999999999919176 ) ;
#32719=DIRECTION ( 'NONE',  ( 0.000000000000000000, 0.000000000000000000, 1.000000000000000000 ) ) ;
#32734=AXIS2_PLACEMENT_3D ( 'NONE', #24217, #5975, #17070 ) ;
#32735=ORIENTED_EDGE ( 'NONE', *, *, #5689, .F. ) ;
#32740=ORIENTED_EDGE ( 'NONE', *, *, #17520, .F. ) ;
#32744=CIRCLE ( 'NONE', #15781, 6.119000000000013095 ) ;
#32758=CARTESIAN_POINT ( 'NONE',  ( -728.8365100919714905, 256.5000000000001705, -199.9999999999890861 ) ) ;
#32761=DIRECTION ( 'NONE',  ( -1.000000000000000000, 0.000000000000000000, 0.000000000000000000 ) ) ;
#32769=LINE ( 'NONE', #19747, #28578 ) ;
#32780=ORIENTED_EDGE ( 'NONE', *, *, #36838, .T. ) ;
#32787=ORIENTED_EDGE ( 'NONE', *, *, #41538, .F. ) ;
#32791=( GEOMETRIC_REPRESENTATION_CONTEXT ( 3 ) GLOBAL_UNCERTAINTY_ASSIGNED_CONTEXT ( ( #40298 ) ) GLOBAL_UNIT_ASSIGNED_CONTEXT ( ( #17635, #3305, #35173 ) ) REPRESENTATION_CONTEXT ( 'NONE', 'WORKASPACE' ) );
#32802=ORIENTED_EDGE ( 'NONE', *, *, #28955, .T. ) ;
#32826=AXIS2_PLACEMENT_3D ( 'NONE', #8578, #37179, #5099 ) ;
#32827=( NAMED_UNIT ( * ) SI_UNIT ( $, .STERADIAN. ) SOLID_ANGLE_UNIT ( ) );
#32846=AXIS2_PLACEMENT_3D ( 'NONE', #33828, #3037, #30352 ) ;
#32866=EDGE_CURVE ( 'NONE', #4510, #27542, #2458, .T. ) ;
#32868=DIRECTION ( 'NONE',  ( 0.000000000000000000, -1.000000000000000000, 0.000000000000000000 ) ) ;
#32895=ORIENTED_EDGE ( 'NONE', *, *, #4622, .F. ) ;
#32906=EDGE_LOOP ( 'NONE', ( #18376, #16490 ) ) ;
#32918=EDGE_LOOP ( 'NONE', ( #24818, #2376 ) ) ;
#32930=CARTESIAN_POINT ( 'NONE',  ( -78.83651009197140525, 260.0000000000000568, -199.9999999999936051 ) ) ;
#32954=CIRCLE ( 'NONE', #21136, 2.749999999999919176 ) ;
#32955=DIRECTION ( 'NONE',  ( -0.000000000000000000, 1.000000000000000000, -0.000000000000000000 ) ) ;
#32979=VECTOR ( 'NONE', #40083, 1000.000000000000000 ) ;
#32982=AXIS2_PLACEMENT_3D ( 'NONE', #42282, #14592, #39286 ) ;
#32983=VERTEX_POINT ( 'NONE', #11933 ) ;
#33005=ORIENTED_EDGE ( 'NONE', *, *, #7197, .T. ) ;
#33037=AXIS2_PLACEMENT_3D ( 'NONE', #22802, #41503, #33881 ) ;
#33049=DIRECTION ( 'NONE',  ( -0.000000000000000000, 1.000000000000000000, -0.000000000000000000 ) ) ;
#33060=CARTESIAN_POINT ( 'NONE',  ( -598.8365100919716042, 260.0000000000001705, -199.9999999999899671 ) ) ;
#33085=DIRECTION ( 'NONE',  ( -0.000000000000000000, 1.000000000000000000, -0.000000000000000000 ) ) ;
#33127=DIRECTION ( 'NONE',  ( 0.000000000000000000, 0.7071067811865474617, 0.7071067811865474617 ) ) ;
#33138=ORIENTED_EDGE ( 'NONE', *, *, #2980, .F. ) ;
#33142=ORIENTED_EDGE ( 'NONE', *, *, #11632, .T. ) ;
#33162=FACE_BOUND ( 'NONE', #44155, .T. ) ;
#33164=ADVANCED_FACE ( 'NONE', ( #30161, #41250 ), #9606, .F. ) ;
#33183=EDGE_CURVE ( 'NONE', #21203, #28948, #16536, .T. ) ;
#33189=CARTESIAN_POINT ( 'NONE',  ( 837.2824899080285377, 256.4999999999998863, -199.9999999999999432 ) ) ;
#33219=VERTEX_POINT ( 'NONE', #29936 ) ;
#33237=EDGE_LOOP ( 'NONE', ( #9224, #18326, #38767, #25900 ) ) ;
#33253=ORIENTED_EDGE ( 'NONE', *, *, #6120, .F. ) ;
#33257=CARTESIAN_POINT ( 'NONE',  ( 571.1634899080285095, 258.0939999999999372, -199.9999999999981526 ) ) ;
#33258=CARTESIAN_POINT ( 'NONE',  ( 181.1634899080285948, 240.0000000000000284, -197.2499999999955662 ) ) ;
#33268=DIRECTION ( 'NONE',  ( -0.000000000000000000, 1.000000000000000000, -0.000000000000000000 ) ) ;
#33343=ORIENTED_EDGE ( 'NONE', *, *, #39725, .F. ) ;
#33349=CIRCLE ( 'NONE', #13448, 8.025000000000003908 ) ;
#33368=FACE_OUTER_BOUND ( 'NONE', #5280, .T. ) ;
#33389=ORIENTED_EDGE ( 'NONE', *, *, #12822, .T. ) ;
#33406=PRODUCT_DEFINITION_FORMATION_WITH_SPECIFIED_SOURCE ( 'ANY', '', #38824, .NOT_KNOWN. ) ;
#33419=CARTESIAN_POINT ( 'NONE',  ( 571.1634899080285095, 256.4999999999999432, -199.9999999999981526 ) ) ;
#33435=VERTEX_POINT ( 'NONE', #13988 ) ;
#33514=CYLINDRICAL_SURFACE ( 'NONE', #36007, 2.749999999999863665 ) ;
#33519=ORIENTED_EDGE ( 'NONE', *, *, #19907, .T. ) ;
#33520=AXIS2_PLACEMENT_3D ( 'NONE', #45388, #24122, #41007 ) ;
#33524=VERTEX_POINT ( 'NONE', #13767 ) ;
#33534=CIRCLE ( 'NONE', #16600, 8.025000000000003908 ) ;
#33554=CARTESIAN_POINT ( 'NONE',  ( -338.8365100919713200, 260.0000000000001137, -199.9999999999917861 ) ) ;
#33560=CARTESIAN_POINT ( 'NONE',  ( -598.8365100919716042, 240.0000000000001705, -197.2499999999901092 ) ) ;
#33562=ORIENTED_EDGE ( 'NONE', *, *, #31441, .T. ) ;
#33564=CIRCLE ( 'NONE', #2570, 2.749999999999891642 ) ;
#33572=VECTOR ( 'NONE', #39550, 1000.000000000000000 ) ;
#33582=AXIS2_PLACEMENT_3D ( 'NONE', #35491, #4328, #43346 ) ;
#33594=CARTESIAN_POINT ( 'NONE',  ( 51.16348990802859475, 256.5000000000000568, -197.2499999999946283 ) ) ;
#33599=CARTESIAN_POINT ( 'NONE',  ( 831.1634899080286232, 256.4999999999998863, -199.9999999999999432 ) ) ;
#33600=DIRECTION ( 'NONE',  ( 0.000000000000000000, 0.000000000000000000, 1.000000000000000000 ) ) ;
#33609=AXIS2_PLACEMENT_3D ( 'NONE', #30177, #36886, #5700 ) ;
#33643=AXIS2_PLACEMENT_3D ( 'NONE', #25541, #39654, #8006 ) ;
#33653=CARTESIAN_POINT ( 'NONE',  ( -208.8365100919714052, 260.0000000000001137, -199.9999999999926956 ) ) ;
#33657=DIRECTION ( 'NONE',  ( -0.000000000000000000, 1.000000000000000000, -0.000000000000000000 ) ) ;
#33666=FACE_OUTER_BOUND ( 'NONE', #10995, .T. ) ;
#33669=EDGE_CURVE ( 'NONE', #34711, #28297, #45538, .T. ) ;
#33673=CIRCLE ( 'NONE', #31466, 2.749999999999842792 ) ;
#33680=CIRCLE ( 'NONE', #1953, 6.118999999999985562 ) ;
#33682=DIRECTION ( 'NONE',  ( -0.000000000000000000, 1.000000000000000000, -0.000000000000000000 ) ) ;
#33686=AXIS2_PLACEMENT_3D ( 'NONE', #17865, #28485, #7946 ) ;
#33693=ORIENTED_EDGE ( 'NONE', *, *, #42741, .F. ) ;
#33706=AXIS2_PLACEMENT_3D ( 'NONE', #4252, #32423, #773 ) ;
#33722=CARTESIAN_POINT ( 'NONE',  ( -78.83651009197140525, 240.0000000000000568, -197.2499999999937756 ) ) ;
#33731=CARTESIAN_POINT ( 'NONE',  ( 701.1634899080286232, 258.0939999999999372, -193.8809999999990623 ) ) ;
#33762=ORIENTED_EDGE ( 'NONE', *, *, #26079, .T. ) ;
#33768=DIRECTION ( 'NONE',  ( 0.000000000000000000, 0.000000000000000000, 1.000000000000000000 ) ) ;
#33777=PRODUCT_DEFINITION ( 'UNKNOWN', '', #33406, #43063 ) ;
#33800=DIRECTION ( 'NONE',  ( 0.000000000000000000, 0.000000000000000000, 1.000000000000000000 ) ) ;
#33807=EDGE_LOOP ( 'NONE', ( #21765, #23045, #1383, #26002 ) ) ;
#33810=AXIS2_PLACEMENT_3D ( 'NONE', #9945, #17107, #30496 ) ;
#33821=DIRECTION ( 'NONE',  ( 0.000000000000000000, 0.000000000000000000, -1.000000000000000000 ) ) ;
#33828=CARTESIAN_POINT ( 'NONE',  ( 51.16348990802859475, 256.5000000000000568, -199.9999999999945146 ) ) ;
#33834=DIRECTION ( 'NONE',  ( -0.000000000000000000, 1.000000000000000000, -0.000000000000000000 ) ) ;
#33836=CARTESIAN_POINT ( 'NONE',  ( -858.8365100919713768, 240.0000000000002274, -199.9999999999881481 ) ) ;
#33847=AXIS2_PLACEMENT_3D ( 'NONE', #12996, #2350, #27522 ) ;
#33881=DIRECTION ( 'NONE',  ( -1.000000000000000000, 0.000000000000000000, 0.000000000000000000 ) ) ;
#33916=EDGE_CURVE ( 'NONE', #36028, #22786, #43321, .T. ) ;
#33922=ORIENTED_EDGE ( 'NONE', *, *, #1789, .T. ) ;
#33945=CARTESIAN_POINT ( 'NONE',  ( -858.8365100919713768, 240.0000000000002274, -197.2499999999882903 ) ) ;
#33965=FACE_OUTER_BOUND ( 'NONE', #35505, .T. ) ;
#33969=ORIENTED_EDGE ( 'NONE', *, *, #14520, .F. ) ;
#33983=CARTESIAN_POINT ( 'NONE',  ( -338.8365100919713200, 260.0000000000001137, -197.2499999999919282 ) ) ;
#34024=VERTEX_POINT ( 'NONE', #344 ) ;
#34090=AXIS2_PLACEMENT_3D ( 'NONE', #42696, #664, #17766 ) ;
#34117=VERTEX_POINT ( 'NONE', #42622 ) ;
#34152=DIRECTION ( 'NONE',  ( 0.000000000000000000, 0.000000000000000000, 1.000000000000000000 ) ) ;
#34183=AXIS2_PLACEMENT_3D ( 'NONE', #25411, #485, #15029 ) ;
#34190=EDGE_CURVE ( 'NONE', #7001, #41246, #5693, .T. ) ;
#34197=VECTOR ( 'NONE', #7265, 1000.000000000000000 ) ;
#34220=CARTESIAN_POINT ( 'NONE',  ( 831.1634899080286232, 239.9999999999998863, -199.9999999999999432 ) ) ;
#34241=DIRECTION ( 'NONE',  ( 0.000000000000000000, 0.000000000000000000, 1.000000000000000000 ) ) ;
#34245=EDGE_CURVE ( 'NONE', #40829, #22852, #36594, .T. ) ;
#34248=AXIS2_PLACEMENT_3D ( 'NONE', #38611, #6281, #10203 ) ;
#34255=CARTESIAN_POINT ( 'NONE',  ( -728.8365100919714905, 260.0000000000001705, -197.2499999999891998 ) ) ;
#34257=ORIENTED_EDGE ( 'NONE', *, *, #29765, .F. ) ;
#34260=DIRECTION ( 'NONE',  ( 0.000000000000000000, 0.000000000000000000, 1.000000000000000000 ) ) ;
#34265=CYLINDRICAL_SURFACE ( 'NONE', #26093, 2.749999999999863665 ) ;
#34286=EDGE_CURVE ( 'NONE', #41197, #8149, #19042, .T. ) ;
#34290=CIRCLE ( 'NONE', #14399, 6.118999999999985562 ) ;
#34293=AXIS2_PLACEMENT_3D ( 'NONE', #27755, #34460, #14130 ) ;
#34313=CONICAL_SURFACE ( 'NONE', #32109, 8.025000000000003908, 0.7853981633974410625 ) ;
#34349=DIRECTION ( 'NONE',  ( -1.880165489482579047E-16, -1.000000000000000000, -0.000000000000000000 ) ) ;
#34351=VERTEX_POINT ( 'NONE', #11878 ) ;
#34366=VECTOR ( 'NONE', #3318, 1000.000000000000000 ) ;
#34385=FACE_OUTER_BOUND ( 'NONE', #39933, .T. ) ;
#34460=DIRECTION ( 'NONE',  ( 1.892425610156518354E-16, 1.000000000000000000, -0.000000000000000000 ) ) ;
#34470=FACE_BOUND ( 'NONE', #20902, .T. ) ;
#34490=EDGE_LOOP ( 'NONE', ( #45398, #15924, #20687, #13018 ) ) ;
#34496=ORIENTED_EDGE ( 'NONE', *, *, #18978, .F. ) ;
#34507=CARTESIAN_POINT ( 'NONE',  ( -879.9999999999992042, 260.0000000000002274, -219.9999999999999716 ) ) ;
#34516=LINE ( 'NONE', #40754, #29711 ) ;
#34520=CARTESIAN_POINT ( 'NONE',  ( 441.1634899080286232, 258.0939999999999372, -199.9999999999972431 ) ) ;
#34544=EDGE_LOOP ( 'NONE', ( #23477, #40201, #41436, #43001 ) ) ;
#34546=CONICAL_SURFACE ( 'NONE', #24211, 8.024999999999948841, 0.7853981633974337351 ) ;
#34568=DIRECTION ( 'NONE',  ( -0.000000000000000000, 1.000000000000000000, -0.000000000000000000 ) ) ;
#34606=ORIENTED_EDGE ( 'NONE', *, *, #39356, .F. ) ;
#34675=CARTESIAN_POINT ( 'NONE',  ( -598.8365100919716042, 260.0000000000001705, -208.0249999999899160 ) ) ;
#34701=DIRECTION ( 'NONE',  ( -0.000000000000000000, 1.000000000000000000, -0.000000000000000000 ) ) ;
#34710=DIRECTION ( 'NONE',  ( 1.892425610156518354E-16, 1.000000000000000000, -0.000000000000000000 ) ) ;
#34711=VERTEX_POINT ( 'NONE', #37720 ) ;
#34724=EDGE_LOOP ( 'NONE', ( #23633, #9773 ) ) ;
#34740=CYLINDRICAL_SURFACE ( 'NONE', #44552, 2.749999999999835687 ) ;
#34775=CARTESIAN_POINT ( 'NONE',  ( 51.16348990802859475, 260.0000000000000568, -199.9999999999945146 ) ) ;
#34793=FACE_OUTER_BOUND ( 'NONE', #22710, .T. ) ;
#34797=EDGE_CURVE ( 'NONE', #30554, #44542, #40425, .T. ) ;
#34801=CIRCLE ( 'NONE', #4549, 2.749999999999919176 ) ;
#34807=CARTESIAN_POINT ( 'NONE',  ( 831.1634899080286232, 259.9999999999998863, -208.0249999999998920 ) ) ;
#34821=ORIENTED_EDGE ( 'NONE', *, *, #16443, .T. ) ;
#34823=EDGE_CURVE ( 'NONE', #3234, #14904, #41149, .T. ) ;
#34835=DIRECTION ( 'NONE',  ( -0.000000000000000000, 1.000000000000000000, -0.000000000000000000 ) ) ;
#34838=CARTESIAN_POINT ( 'NONE',  ( 831.1634899080286232, 258.0939999999998804, -206.1189999999999429 ) ) ;
#34846=ADVANCED_FACE ( 'NONE', ( #31696 ), #8712, .F. ) ;
#34861=EDGE_CURVE ( 'NONE', #10866, #15586, #8148, .T. ) ;
#34881=EDGE_CURVE ( 'NONE', #27295, #31800, #45571, .T. ) ;
#34905=ADVANCED_FACE ( 'NONE', ( #22211 ), #32161, .F. ) ;
#34916=FACE_BOUND ( 'NONE', #3035, .T. ) ;
#34949=DIRECTION ( 'NONE',  ( 0.000000000000000000, 0.000000000000000000, 1.000000000000000000 ) ) ;
#34961=CARTESIAN_POINT ( 'NONE',  ( -598.8365100919716042, 260.0000000000001705, -191.9749999999900183 ) ) ;
#34982=ORIENTED_EDGE ( 'NONE', *, *, #24620, .F. ) ;
#34991=EDGE_LOOP ( 'NONE', ( #30655, #36824, #44655, #36727 ) ) ;
#35007=AXIS2_PLACEMENT_3D ( 'NONE', #3586, #10491, #35211 ) ;
#35014=CARTESIAN_POINT ( 'NONE',  ( -728.8365100919714905, 260.0000000000001705, -191.9749999999891372 ) ) ;
#35039=EDGE_LOOP ( 'NONE', ( #15240, #42572, #16362, #45658 ) ) ;
#35045=ORIENTED_EDGE ( 'NONE', *, *, #1009, .F. ) ;
#35051=AXIS2_PLACEMENT_3D ( 'NONE', #29815, #43895, #8807 ) ;
#35067=DIRECTION ( 'NONE',  ( -0.000000000000000000, 1.000000000000000000, -0.000000000000000000 ) ) ;
#35106=DIRECTION ( 'NONE',  ( 0.000000000000000000, 0.000000000000000000, 1.000000000000000000 ) ) ;
#35107=ORIENTED_EDGE ( 'NONE', *, *, #28955, .F. ) ;
#35122=EDGE_CURVE ( 'NONE', #32688, #35282, #44840, .T. ) ;
#35131=CARTESIAN_POINT ( 'NONE',  ( -728.8365100919714905, 256.5000000000001705, -199.9999999999890861 ) ) ;
#35146=FACE_BOUND ( 'NONE', #23224, .T. ) ;
#35154=CYLINDRICAL_SURFACE ( 'NONE', #15951, 2.749999999999835687 ) ;
#35157=EDGE_LOOP ( 'NONE', ( #31873, #15840 ) ) ;
#35170=CIRCLE ( 'NONE', #45505, 6.119000000000013095 ) ;
#35172=ORIENTED_EDGE ( 'NONE', *, *, #3488, .F. ) ;
#35173=( NAMED_UNIT ( * ) SI_UNIT ( $, .STERADIAN. ) SOLID_ANGLE_UNIT ( ) );
#35177=EDGE_CURVE ( 'NONE', #34117, #41429, #15524, .T. ) ;
#35193=FACE_OUTER_BOUND ( 'NONE', #2318, .T. ) ;
#35196=CARTESIAN_POINT ( 'NONE',  ( -728.8365100919714905, 260.0000000000001705, -208.0249999999890349 ) ) ;
#35211=DIRECTION ( 'NONE',  ( 0.000000000000000000, 0.000000000000000000, 1.000000000000000000 ) ) ;
#35282=VERTEX_POINT ( 'NONE', #37197 ) ;
#35298=CARTESIAN_POINT ( 'NONE',  ( -468.8365100919714337, 240.0000000000001421, -199.9999999999908766 ) ) ;
#35305=ORIENTED_EDGE ( 'NONE', *, *, #32866, .F. ) ;
#35327=ORIENTED_EDGE ( 'NONE', *, *, #37858, .T. ) ;
#35345=CARTESIAN_POINT ( 'NONE',  ( -598.8365100919716042, 260.0000000000001705, -202.7499999999898250 ) ) ;
#35350=EDGE_CURVE ( 'NONE', #29032, #17994, #13123, .T. ) ;
#35351=ORIENTED_EDGE ( 'NONE', *, *, #10512, .F. ) ;
#35370=ADVANCED_FACE ( 'NONE', ( #9027 ), #33514, .F. ) ;
#35371=CARTESIAN_POINT ( 'NONE',  ( 4.541821464375645154E-14, 240.0000000000000568, 0.000000000000000000 ) ) ;
#35379=ORIENTED_EDGE ( 'NONE', *, *, #16508, .F. ) ;
#35397=ORIENTED_EDGE ( 'NONE', *, *, #13311, .T. ) ;
#35403=DIRECTION ( 'NONE',  ( -0.000000000000000000, 1.000000000000000000, -0.000000000000000000 ) ) ;
#35404=FACE_OUTER_BOUND ( 'NONE', #45214, .T. ) ;
#35438=ORIENTED_EDGE ( 'NONE', *, *, #35122, .T. ) ;
#35446=ORIENTED_EDGE ( 'NONE', *, *, #26959, .F. ) ;
#35460=CARTESIAN_POINT ( 'NONE',  ( 701.1634899080286232, 259.9999999999999432, -191.9749999999990848 ) ) ;
#35484=DIRECTION ( 'NONE',  ( -1.000000000000000000, 0.000000000000000000, 0.000000000000000000 ) ) ;
#35491=CARTESIAN_POINT ( 'NONE',  ( 181.1634899080285948, 260.0000000000000000, -199.9999999999953957 ) ) ;
#35494=ADVANCED_FACE ( 'NONE', ( #30742 ), #27277, .F. ) ;
#35505=EDGE_LOOP ( 'NONE', ( #19109, #9682, #1201, #28468 ) ) ;
#35586=EDGE_CURVE ( 'NONE', #45239, #27745, #6014, .T. ) ;
#35587=DIRECTION ( 'NONE',  ( 0.000000000000000000, 0.000000000000000000, 1.000000000000000000 ) ) ;
#35611=CARTESIAN_POINT ( 'NONE',  ( 51.16348990802859475, 260.0000000000000568, -202.7499999999943441 ) ) ;
#35620=ORIENTED_EDGE ( 'NONE', *, *, #36196, .T. ) ;
#35627=CARTESIAN_POINT ( 'NONE',  ( 571.1634899080285095, 259.9999999999999432, -202.7499999999980105 ) ) ;
#35632=DIRECTION ( 'NONE',  ( -0.000000000000000000, 1.000000000000000000, -0.000000000000000000 ) ) ;
#35639=CARTESIAN_POINT ( 'NONE',  ( 577.2824899080285377, 256.4999999999999432, -199.9999999999981526 ) ) ;
#35647=DIRECTION ( 'NONE',  ( -0.000000000000000000, 1.000000000000000000, -0.000000000000000000 ) ) ;
#35660=DIRECTION ( 'NONE',  ( -0.000000000000000000, 1.000000000000000000, -0.000000000000000000 ) ) ;
#35664=ORIENTED_EDGE ( 'NONE', *, *, #9997, .F. ) ;
#35677=ORIENTED_EDGE ( 'NONE', *, *, #42760, .T. ) ;
#35680=AXIS2_PLACEMENT_3D ( 'NONE', #7492, #35647, #12318 ) ;
#35681=ORIENTED_EDGE ( 'NONE', *, *, #29360, .F. ) ;
#35686=DIRECTION ( 'NONE',  ( -0.000000000000000000, 1.000000000000000000, -0.000000000000000000 ) ) ;
#35696=CYLINDRICAL_SURFACE ( 'NONE', #14561, 2.749999999999835687 ) ;
#35703=ADVANCED_FACE ( 'NONE', ( #33965 ), #13421, .F. ) ;
#35720=ADVANCED_FACE ( 'NONE', ( #38360 ), #6706, .F. ) ;
#35726=VERTEX_POINT ( 'NONE', #18025 ) ;
#35800=EDGE_LOOP ( 'NONE', ( #11319, #11674 ) ) ;
#35824=DIRECTION ( 'NONE',  ( -0.000000000000000000, 1.000000000000000000, -0.000000000000000000 ) ) ;
#35832=DIRECTION ( 'NONE',  ( 0.000000000000000000, 0.000000000000000000, 1.000000000000000000 ) ) ;
#35841=FACE_BOUND ( 'NONE', #29872, .T. ) ;
#35850=ORIENTED_EDGE ( 'NONE', *, *, #10607, .F. ) ;
#35859=CIRCLE ( 'NONE', #21848, 6.118999999999985562 ) ;
#35875=AXIS2_PLACEMENT_3D ( 'NONE', #9227, #19387, #12242 ) ;
#35895=VECTOR ( 'NONE', #30815, 1000.000000000000000 ) ;
#35919=ORIENTED_EDGE ( 'NONE', *, *, #5793, .F. ) ;
#35942=CARTESIAN_POINT ( 'NONE',  ( -598.8365100919716042, 256.5000000000001705, -199.9999999999899671 ) ) ;
#36004=ORIENTED_EDGE ( 'NONE', *, *, #3388, .F. ) ;
#36007=AXIS2_PLACEMENT_3D ( 'NONE', #18992, #33085, #1863 ) ;
#36014=EDGE_CURVE ( 'NONE', #30790, #18371, #38249, .T. ) ;
#36025=DIRECTION ( 'NONE',  ( 0.000000000000000000, 0.000000000000000000, 1.000000000000000000 ) ) ;
#36028=VERTEX_POINT ( 'NONE', #6934 ) ;
#36065=( NAMED_UNIT ( * ) PLANE_ANGLE_UNIT ( ) SI_UNIT ( $, .RADIAN. ) );
#36072=DIRECTION ( 'NONE',  ( -0.000000000000000000, 1.000000000000000000, -0.000000000000000000 ) ) ;
#36123=CARTESIAN_POINT ( 'NONE',  ( 831.1634899080286232, 256.4999999999998863, -199.9999999999999432 ) ) ;
#36132=CARTESIAN_POINT ( 'NONE',  ( -468.8365100919714337, 258.0940000000001646, -199.9999999999908766 ) ) ;
#36148=ORIENTED_EDGE ( 'NONE', *, *, #32371, .T. ) ;
#36154=DIRECTION ( 'NONE',  ( 0.000000000000000000, -1.000000000000000000, 0.000000000000000000 ) ) ;
#36162=DIRECTION ( 'NONE',  ( -0.000000000000000000, 1.000000000000000000, -0.000000000000000000 ) ) ;
#36168=DIRECTION ( 'NONE',  ( -0.000000000000000000, 1.000000000000000000, -0.000000000000000000 ) ) ;
#36186=VERTEX_POINT ( 'NONE', #37818 ) ;
#36196=EDGE_CURVE ( 'NONE', #26360, #15531, #6167, .T. ) ;
#36209=CARTESIAN_POINT ( 'NONE',  ( -78.83651009197140525, 260.0000000000000568, -202.7499999999934346 ) ) ;
#36216=DIRECTION ( 'NONE',  ( -0.000000000000000000, 1.000000000000000000, -0.000000000000000000 ) ) ;
#36217=EDGE_CURVE ( 'NONE', #2736, #38472, #45447, .T. ) ;
#36223=DIRECTION ( 'NONE',  ( 8.659560562354932858E-17, 0.7071067811865474617, -0.7071067811865474617 ) ) ;
#36248=ADVANCED_FACE ( 'NONE', ( #31106 ), #13807, .F. ) ;
#36258=ORIENTED_EDGE ( 'NONE', *, *, #24682, .F. ) ;
#36263=DIRECTION ( 'NONE',  ( 0.000000000000000000, 0.000000000000000000, 1.000000000000000000 ) ) ;
#36281=ADVANCED_FACE ( 'NONE', ( #10324 ), #34546, .F. ) ;
#36327=VECTOR ( 'NONE', #13275, 1000.000000000000000 ) ;
#36346=VECTOR ( 'NONE', #20698, 1000.000000000000000 ) ;
#36387=CARTESIAN_POINT ( 'NONE',  ( 441.1634899080286232, 239.9999999999999716, -199.9999999999972431 ) ) ;
#36406=ORIENTED_EDGE ( 'NONE', *, *, #38814, .F. ) ;
#36419=ORIENTED_EDGE ( 'NONE', *, *, #13993, .T. ) ;
#36445=AXIS2_PLACEMENT_3D ( 'NONE', #18796, #15337, #39832 ) ;
#36458=CONICAL_SURFACE ( 'NONE', #13614, 8.024999999999948841, 0.7853981633974337351 ) ;
#36461=DIRECTION ( 'NONE',  ( -0.000000000000000000, 1.000000000000000000, -0.000000000000000000 ) ) ;
#36476=ORIENTED_EDGE ( 'NONE', *, *, #43051, .F. ) ;
#36478=EDGE_CURVE ( 'NONE', #26915, #34024, #18191, .T. ) ;
#36508=DIRECTION ( 'NONE',  ( 1.892425610156518354E-16, 1.000000000000000000, -0.000000000000000000 ) ) ;
#36553=DIRECTION ( 'NONE',  ( -0.000000000000000000, 1.000000000000000000, -0.000000000000000000 ) ) ;
#36558=EDGE_CURVE ( 'NONE', #16670, #12174, #30117, .T. ) ;
#36583=DIRECTION ( 'NONE',  ( 0.000000000000000000, 0.000000000000000000, 1.000000000000000000 ) ) ;
#36594=LINE ( 'NONE', #40725, #31518 ) ;
#36613=CARTESIAN_POINT ( 'NONE',  ( 571.1634899080285095, 259.9999999999999432, -191.9749999999982037 ) ) ;
#36626=LINE ( 'NONE', #18402, #39325 ) ;
#36638=AXIS2_PLACEMENT_3D ( 'NONE', #44501, #23242, #29960 ) ;
#36655=AXIS2_PLACEMENT_3D ( 'NONE', #433, #14536, #13842 ) ;
#36701=VERTEX_POINT ( 'NONE', #32266 ) ;
#36706=CARTESIAN_POINT ( 'NONE',  ( -598.8365100919716042, 260.0000000000001705, -208.0249999999899160 ) ) ;
#36719=AXIS2_PLACEMENT_3D ( 'NONE', #31419, #12961, #20105 ) ;
#36721=DIRECTION ( 'NONE',  ( 8.659560562354869996E-17, 0.7071067811865526798, -0.7071067811865423547 ) ) ;
#36727=ORIENTED_EDGE ( 'NONE', *, *, #23804, .T. ) ;
#36773=VERTEX_POINT ( 'NONE', #4322 ) ;
#36804=LINE ( 'NONE', #44406, #38025 ) ;
#36816=EDGE_CURVE ( 'NONE', #31071, #18371, #37926, .T. ) ;
#36824=ORIENTED_EDGE ( 'NONE', *, *, #21615, .F. ) ;
#36830=DIRECTION ( 'NONE',  ( 0.000000000000000000, 0.7071067811865578978, 0.7071067811865372477 ) ) ;
#36838=EDGE_CURVE ( 'NONE', #22371, #6808, #27947, .T. ) ;
#36856=ADVANCED_FACE ( 'NONE', ( #30533 ), #27307, .F. ) ;
#36865=EDGE_LOOP ( 'NONE', ( #4555, #17851 ) ) ;
#36872=ORIENTED_EDGE ( 'NONE', *, *, #12533, .T. ) ;
#36886=DIRECTION ( 'NONE',  ( -0.000000000000000000, 1.000000000000000000, -0.000000000000000000 ) ) ;
#36895=CARTESIAN_POINT ( 'NONE',  ( -78.83651009197140525, 260.0000000000000568, -206.1189999999936049 ) ) ;
#36919=EDGE_LOOP ( 'NONE', ( #24028, #34496 ) ) ;
#36925=DIRECTION ( 'NONE',  ( 0.000000000000000000, -0.000000000000000000, -1.000000000000000000 ) ) ;
#36991=DIRECTION ( 'NONE',  ( -0.000000000000000000, 1.000000000000000000, -0.000000000000000000 ) ) ;
#36994=ORIENTED_EDGE ( 'NONE', *, *, #20363, .T. ) ;
#37061=DIRECTION ( 'NONE',  ( 1.892425610156518354E-16, 1.000000000000000000, -0.000000000000000000 ) ) ;
#37083=ORIENTED_EDGE ( 'NONE', *, *, #15333, .F. ) ;
#37105=DIRECTION ( 'NONE',  ( -0.000000000000000000, 1.000000000000000000, -0.000000000000000000 ) ) ;
#37110=FACE_OUTER_BOUND ( 'NONE', #33237, .T. ) ;
#37121=AXIS2_PLACEMENT_3D ( 'NONE', #26502, #2015, #40603 ) ;
#37162=CARTESIAN_POINT ( 'NONE',  ( 51.16348990802859475, 260.0000000000000568, -199.9999999999945146 ) ) ;
#37179=DIRECTION ( 'NONE',  ( -0.000000000000000000, 1.000000000000000000, -0.000000000000000000 ) ) ;
#37183=CIRCLE ( 'NONE', #23156, 8.025000000000003908 ) ;
#37197=CARTESIAN_POINT ( 'NONE',  ( -728.8365100919714905, 256.5000000000001705, -202.7499999999890008 ) ) ;
#37216=CARTESIAN_POINT ( 'NONE',  ( -338.8365100919713200, 260.0000000000001137, -199.9999999999917861 ) ) ;
#37222=CIRCLE ( 'NONE', #4797, 6.119000000000013095 ) ;
#37239=CARTESIAN_POINT ( 'NONE',  ( -78.83651009197140525, 256.5000000000000568, -199.9999999999936051 ) ) ;
#37245=DIRECTION ( 'NONE',  ( -0.000000000000000000, 1.000000000000000000, -0.000000000000000000 ) ) ;
#37255=CIRCLE ( 'NONE', #1841, 6.118999999999985562 ) ;
#37280=LINE ( 'NONE', #19733, #37372 ) ;
#37287=FACE_OUTER_BOUND ( 'NONE', #18653, .T. ) ;
#37289=CARTESIAN_POINT ( 'NONE',  ( 701.1634899080286232, 256.4999999999999432, -199.9999999999990337 ) ) ;
#37290=CARTESIAN_POINT ( 'NONE',  ( 701.1634899080286232, 256.4999999999999432, -199.9999999999990337 ) ) ;
#37321=DIRECTION ( 'NONE',  ( 0.000000000000000000, -1.000000000000000000, 0.000000000000000000 ) ) ;
#37336=CONICAL_SURFACE ( 'NONE', #15207, 8.024999999999948841, 0.7853981633974337351 ) ;
#37346=DIRECTION ( 'NONE',  ( 0.000000000000000000, 0.000000000000000000, 1.000000000000000000 ) ) ;
#37353=ORIENTED_EDGE ( 'NONE', *, *, #30641, .F. ) ;
#37370=EDGE_LOOP ( 'NONE', ( #36476, #38012, #39406, #8552 ) ) ;
#37372=VECTOR ( 'NONE', #16266, 1000.000000000000114 ) ;
#37382=VECTOR ( 'NONE', #14066, 1000.000000000000000 ) ;
#37415=CARTESIAN_POINT ( 'NONE',  ( 441.1634899080286232, 259.9999999999999432, -199.9999999999972431 ) ) ;
#37434=DIRECTION ( 'NONE',  ( 1.892425610156518354E-16, 1.000000000000000000, -0.000000000000000000 ) ) ;
#37485=CARTESIAN_POINT ( 'NONE',  ( 831.1634899080286232, 239.9999999999998863, -197.2500000000000853 ) ) ;
#37494=ORIENTED_EDGE ( 'NONE', *, *, #32600, .T. ) ;
#37510=FACE_OUTER_BOUND ( 'NONE', #34991, .T. ) ;
#37518=CARTESIAN_POINT ( 'NONE',  ( -598.8365100919716042, 240.0000000000001705, -202.7499999999898250 ) ) ;
#37529=DIRECTION ( 'NONE',  ( 1.892425610156518354E-16, 1.000000000000000000, -0.000000000000000000 ) ) ;
#37544=EDGE_LOOP ( 'NONE', ( #32415, #32034, #12457, #40682 ) ) ;
#37550=ORIENTED_EDGE ( 'NONE', *, *, #18226, .F. ) ;
#37574=DIRECTION ( 'NONE',  ( 0.000000000000000000, 0.000000000000000000, 1.000000000000000000 ) ) ;
#37578=VERTEX_POINT ( 'NONE', #1180 ) ;
#37582=CARTESIAN_POINT ( 'NONE',  ( 181.1634899080285948, 260.0000000000000000, -199.9999999999953957 ) ) ;
#37606=FACE_BOUND ( 'NONE', #37970, .T. ) ;
#37634=CARTESIAN_POINT ( 'NONE',  ( -858.8365100919713768, 260.0000000000002274, -199.9999999999881481 ) ) ;
#37646=DIRECTION ( 'NONE',  ( -0.000000000000000000, 1.000000000000000000, -0.000000000000000000 ) ) ;
#37651=EDGE_CURVE ( 'NONE', #8247, #18328, #14834, .T. ) ;
#37669=EDGE_LOOP ( 'NONE', ( #18830, #12172, #11287, #41381 ) ) ;
#37704=LINE ( 'NONE', #1903, #2538 ) ;
#37720=CARTESIAN_POINT ( 'NONE',  ( 51.16348990802859475, 258.0940000000000509, -206.1189999999945144 ) ) ;
#37738=ORIENTED_EDGE ( 'NONE', *, *, #29360, .T. ) ;
#37741=LINE ( 'NONE', #6092, #35895 ) ;
#37759=CARTESIAN_POINT ( 'NONE',  ( -879.9999999999992042, 260.0000000000002274, -219.9999999999999716 ) ) ;
#37780=CARTESIAN_POINT ( 'NONE',  ( 51.16348990802859475, 258.0940000000000509, -199.9999999999945146 ) ) ;
#37818=CARTESIAN_POINT ( 'NONE',  ( 571.1634899080285095, 256.4999999999999432, -193.8809999999981528 ) ) ;
#37840=ORIENTED_EDGE ( 'NONE', *, *, #26922, .T. ) ;
#37841=ORIENTED_EDGE ( 'NONE', *, *, #18488, .F. ) ;
#37852=CARTESIAN_POINT ( 'NONE',  ( -208.8365100919714052, 260.0000000000001137, -202.7499999999925251 ) ) ;
#37858=EDGE_CURVE ( 'NONE', #36186, #6776, #23508, .T. ) ;
#37877=CARTESIAN_POINT ( 'NONE',  ( 181.1634899080285948, 260.0000000000000000, -199.9999999999953957 ) ) ;
#37891=EDGE_CURVE ( 'NONE', #10815, #25509, #41128, .T. ) ;
#37926=LINE ( 'NONE', #11918, #41205 ) ;
#37970=EDGE_LOOP ( 'NONE', ( #26818, #23143 ) ) ;
#37993=DIRECTION ( 'NONE',  ( 0.000000000000000000, 0.000000000000000000, 1.000000000000000000 ) ) ;
#38001=FACE_BOUND ( 'NONE', #34724, .T. ) ;
#38007=CIRCLE ( 'NONE', #18098, 2.749999999999808153 ) ;
#38012=ORIENTED_EDGE ( 'NONE', *, *, #28976, .T. ) ;
#38021=CIRCLE ( 'NONE', #43896, 8.024999999999948841 ) ;
#38025=VECTOR ( 'NONE', #12761, 1000.000000000000000 ) ;
#38028=EDGE_LOOP ( 'NONE', ( #20400, #24639, #8315, #5764 ) ) ;
#38048=VERTEX_POINT ( 'NONE', #33731 ) ;
#38077=CARTESIAN_POINT ( 'NONE',  ( 441.1634899080286232, 258.0939999999999372, -206.1189999999972144 ) ) ;
#38078=EDGE_LOOP ( 'NONE', ( #29443, #45057, #33389, #36148 ) ) ;
#38083=VECTOR ( 'NONE', #26518, 1000.000000000000000 ) ;
#38095=CARTESIAN_POINT ( 'NONE',  ( -879.9999999999992042, 260.0000000000002274, -219.9999999999999716 ) ) ;
#38109=CIRCLE ( 'NONE', #18207, 6.118999999999985562 ) ;
#38148=VECTOR ( 'NONE', #36553, 1000.000000000000000 ) ;
#38151=AXIS2_PLACEMENT_3D ( 'NONE', #12797, #29673, #40748 ) ;
#38156=ADVANCED_FACE ( 'NONE', ( #29806 ), #22797, .F. ) ;
#38179=VECTOR ( 'NONE', #9322, 1000.000000000000000 ) ;
#38183=EDGE_LOOP ( 'NONE', ( #26719, #5572 ) ) ;
#38212=CARTESIAN_POINT ( 'NONE',  ( -338.8365100919713200, 240.0000000000001137, -199.9999999999917861 ) ) ;
#38216=FACE_OUTER_BOUND ( 'NONE', #12284, .T. ) ;
#38230=PLANE ( 'NONE',  #329 ) ;
#38249=CIRCLE ( 'NONE', #8024, 8.025000000000003908 ) ;
#38265=EDGE_CURVE ( 'NONE', #40312, #18427, #42720, .T. ) ;
#38360=FACE_OUTER_BOUND ( 'NONE', #31299, .T. ) ;
#38393=DIRECTION ( 'NONE',  ( 0.000000000000000000, 0.000000000000000000, 1.000000000000000000 ) ) ;
#38432=CARTESIAN_POINT ( 'NONE',  ( 571.1634899080285095, 256.4999999999999432, -197.2499999999982379 ) ) ;
#38435=CARTESIAN_POINT ( 'NONE',  ( -208.8365100919714052, 260.0000000000001137, -206.1189999999926954 ) ) ;
#38463=ORIENTED_EDGE ( 'NONE', *, *, #21597, .T. ) ;
#38472=VERTEX_POINT ( 'NONE', #31629 ) ;
#38490=CARTESIAN_POINT ( 'NONE',  ( -879.9999999999992042, 240.0000000000002274, -179.9999999999999716 ) ) ;
#38501=CIRCLE ( 'NONE', #15656, 6.118999999999985562 ) ;
#38525=ORIENTED_EDGE ( 'NONE', *, *, #35177, .F. ) ;
#38539=CARTESIAN_POINT ( 'NONE',  ( -598.8365100919716042, 260.0000000000001705, -197.2499999999901092 ) ) ;
#38580=CARTESIAN_POINT ( 'NONE',  ( -468.8365100919714337, 260.0000000000001705, -199.9999999999908766 ) ) ;
#38581=ORIENTED_EDGE ( 'NONE', *, *, #22188, .F. ) ;
#38599=CARTESIAN_POINT ( 'NONE',  ( -598.8365100919716042, 256.5000000000001705, -206.1189999999899385 ) ) ;
#38609=CARTESIAN_POINT ( 'NONE',  ( -468.8365100919714337, 260.0000000000001705, -206.1189999999908764 ) ) ;
#38611=CARTESIAN_POINT ( 'NONE',  ( -208.8365100919714052, 240.0000000000000853, -199.9999999999926956 ) ) ;
#38625=AXIS2_PLACEMENT_3D ( 'NONE', #30933, #40867, #23521 ) ;
#38631=ORIENTED_EDGE ( 'NONE', *, *, #38265, .T. ) ;
#38642=AXIS2_PLACEMENT_3D ( 'NONE', #38212, #30580, #45137 ) ;
#38664=CARTESIAN_POINT ( 'NONE',  ( 831.1634899080286232, 258.0939999999998804, -193.8809999999999718 ) ) ;
#38699=EDGE_LOOP ( 'NONE', ( #32679, #25860, #12660, #3659 ) ) ;
#38713=DIRECTION ( 'NONE',  ( 0.000000000000000000, 0.000000000000000000, 1.000000000000000000 ) ) ;
#38714=CARTESIAN_POINT ( 'NONE',  ( 571.1634899080285095, 259.9999999999999432, -197.2499999999982947 ) ) ;
#38722=DIRECTION ( 'NONE',  ( -0.000000000000000000, 1.000000000000000000, -0.000000000000000000 ) ) ;
#38728=DIRECTION ( 'NONE',  ( 0.000000000000000000, 0.000000000000000000, 1.000000000000000000 ) ) ;
#38734=ADVANCED_FACE ( 'NONE', ( #37510 ), #8828, .F. ) ;
#38736=DIRECTION ( 'NONE',  ( -0.000000000000000000, 1.000000000000000000, -0.000000000000000000 ) ) ;
#38752=DIRECTION ( 'NONE',  ( 8.659560562354807133E-17, 0.7071067811865578978, -0.7071067811865372477 ) ) ;
#38767=ORIENTED_EDGE ( 'NONE', *, *, #18268, .T. ) ;
#38785=DIRECTION ( 'NONE',  ( 0.000000000000000000, -1.000000000000000000, 0.000000000000000000 ) ) ;
#38787=ADVANCED_FACE ( 'NONE', ( #30340 ), #44432, .F. ) ;
#38804=AXIS2_PLACEMENT_3D ( 'NONE', #3560, #35403, #3774 ) ;
#38814=EDGE_CURVE ( 'NONE', #13375, #3205, #40551, .T. ) ;
#38819=ORIENTED_EDGE ( 'NONE', *, *, #28972, .T. ) ;
#38824=PRODUCT ( 'Lower Fixed Bed Shear Blade', 'Lower Fixed Bed Shear Blade', '', ( #18215 ) ) ;
#38837=EDGE_LOOP ( 'NONE', ( #42798, #7523, #44070, #1251 ) ) ;
#38841=LINE ( 'NONE', #9566, #42501 ) ;
#38857=ADVANCED_FACE ( 'NONE', ( #10241 ), #41273, .F. ) ;
#38879=AXIS2_PLACEMENT_3D ( 'NONE', #7835, #11521, #32308 ) ;
#38890=CONICAL_SURFACE ( 'NONE', #36638, 8.025000000000003908, 0.7853981633974482790 ) ;
#38911=VECTOR ( 'NONE', #36223, 1000.000000000000114 ) ;
#38912=CARTESIAN_POINT ( 'NONE',  ( 51.16348990802859475, 260.0000000000000568, -206.1189999999945428 ) ) ;
#38938=ORIENTED_EDGE ( 'NONE', *, *, #24678, .T. ) ;
#38989=FACE_OUTER_BOUND ( 'NONE', #21017, .T. ) ;
#38991=EDGE_LOOP ( 'NONE', ( #19158, #23980 ) ) ;
#39000=ORIENTED_EDGE ( 'NONE', *, *, #40778, .F. ) ;
#39091=FACE_BOUND ( 'NONE', #42430, .T. ) ;
#39100=ORIENTED_EDGE ( 'NONE', *, *, #12287, .T. ) ;
#39124=CARTESIAN_POINT ( 'NONE',  ( -208.8365100919714052, 240.0000000000000853, -202.7499999999925251 ) ) ;
#39126=ORIENTED_EDGE ( 'NONE', *, *, #3842, .F. ) ;
#39139=DIRECTION ( 'NONE',  ( -1.000000000000000000, 0.000000000000000000, 0.000000000000000000 ) ) ;
#39210=CARTESIAN_POINT ( 'NONE',  ( 311.1634899080286232, 256.5000000000000000, -193.8809999999963338 ) ) ;
#39224=ORIENTED_EDGE ( 'NONE', *, *, #10590, .T. ) ;
#39271=DIRECTION ( 'NONE',  ( -0.000000000000000000, 1.000000000000000000, -0.000000000000000000 ) ) ;
#39281=VERTEX_POINT ( 'NONE', #10703 ) ;
#39286=DIRECTION ( 'NONE',  ( 0.000000000000000000, -0.000000000000000000, -1.000000000000000000 ) ) ;
#39301=AXIS2_PLACEMENT_3D ( 'NONE', #35639, #39826, #3787 ) ;
#39304=CARTESIAN_POINT ( 'NONE',  ( 181.1634899080285948, 258.0939999999999941, -206.1189999999954239 ) ) ;
#39311=DIRECTION ( 'NONE',  ( 0.000000000000000000, 0.000000000000000000, 1.000000000000000000 ) ) ;
#39325=VECTOR ( 'NONE', #43328, 1000.000000000000000 ) ;
#39327=CARTESIAN_POINT ( 'NONE',  ( -598.8365100919716042, 240.0000000000001705, -199.9999999999899671 ) ) ;
#39356=EDGE_CURVE ( 'NONE', #18371, #30790, #22632, .T. ) ;
#39359=DIRECTION ( 'NONE',  ( -0.000000000000000000, 1.000000000000000000, -0.000000000000000000 ) ) ;
#39368=ADVANCED_FACE ( 'NONE', ( #35404 ), #3775, .F. ) ;
#39375=AXIS2_PLACEMENT_3D ( 'NONE', #33189, #37321, #19100 ) ;
#39376=DIRECTION ( 'NONE',  ( 0.000000000000000000, 0.000000000000000000, 1.000000000000000000 ) ) ;
#39398=ORIENTED_EDGE ( 'NONE', *, *, #4128, .F. ) ;
#39404=FACE_OUTER_BOUND ( 'NONE', #17737, .T. ) ;
#39406=ORIENTED_EDGE ( 'NONE', *, *, #22762, .T. ) ;
#39408=CYLINDRICAL_SURFACE ( 'NONE', #5613, 6.118999999999985562 ) ;
#39411=VECTOR ( 'NONE', #15998, 999.9999999999998863 ) ;
#39418=DIRECTION ( 'NONE',  ( 0.000000000000000000, 0.000000000000000000, 1.000000000000000000 ) ) ;
#39452=AXIS2_PLACEMENT_3D ( 'NONE', #16065, #32955, #44007 ) ;
#39474=DIRECTION ( 'NONE',  ( -0.000000000000000000, 1.000000000000000000, -0.000000000000000000 ) ) ;
#39478=DIRECTION ( 'NONE',  ( -0.000000000000000000, 1.000000000000000000, -0.000000000000000000 ) ) ;
#39504=CIRCLE ( 'NONE', #41697, 6.118999999999985562 ) ;
#39520=AXIS2_PLACEMENT_3D ( 'NONE', #3357, #2665, #13758 ) ;
#39521=CIRCLE ( 'NONE', #23289, 6.118999999999985562 ) ;
#39537=AXIS2_PLACEMENT_3D ( 'NONE', #17652, #35632, #31263 ) ;
#39550=DIRECTION ( 'NONE',  ( 0.000000000000000000, 0.7071067811865526798, 0.7071067811865423547 ) ) ;
#39576=ORIENTED_EDGE ( 'NONE', *, *, #6649, .T. ) ;
#39577=CIRCLE ( 'NONE', #15242, 2.749999999999919176 ) ;
#39584=EDGE_CURVE ( 'NONE', #32411, #12435, #30287, .T. ) ;
#39593=DIRECTION ( 'NONE',  ( -0.000000000000000000, 1.000000000000000000, -0.000000000000000000 ) ) ;
#39594=ORIENTED_EDGE ( 'NONE', *, *, #25287, .T. ) ;
#39599=FACE_BOUND ( 'NONE', #27214, .T. ) ;
#39619=LINE ( 'NONE', #18812, #1178 ) ;
#39633=EDGE_CURVE ( 'NONE', #29759, #14400, #3461, .T. ) ;
#39654=DIRECTION ( 'NONE',  ( 1.892425610156518354E-16, 1.000000000000000000, -0.000000000000000000 ) ) ;
#39658=FACE_OUTER_BOUND ( 'NONE', #29392, .T. ) ;
#39664=DIRECTION ( 'NONE',  ( 0.000000000000000000, 0.000000000000000000, 1.000000000000000000 ) ) ;
#39680=ORIENTED_EDGE ( 'NONE', *, *, #17880, .F. ) ;
#39725=EDGE_CURVE ( 'NONE', #42507, #25509, #29288, .T. ) ;
#39746=ADVANCED_FACE ( 'NONE', ( #40262 ), #32246, .F. ) ;
#39759=ORIENTED_EDGE ( 'NONE', *, *, #13735, .T. ) ;
#39761=ORIENTED_EDGE ( 'NONE', *, *, #109, .F. ) ;
#39765=DIRECTION ( 'NONE',  ( 0.000000000000000000, 0.000000000000000000, 1.000000000000000000 ) ) ;
#39826=DIRECTION ( 'NONE',  ( 0.000000000000000000, -1.000000000000000000, 0.000000000000000000 ) ) ;
#39829=CARTESIAN_POINT ( 'NONE',  ( 701.1634899080286232, 259.9999999999999432, -208.0249999999989825 ) ) ;
#39832=DIRECTION ( 'NONE',  ( 0.000000000000000000, 0.000000000000000000, 1.000000000000000000 ) ) ;
#39848=EDGE_LOOP ( 'NONE', ( #13531, #25457, #13130, #19269 ) ) ;
#39875=CARTESIAN_POINT ( 'NONE',  ( 181.1634899080285948, 240.0000000000000284, -202.7499999999952536 ) ) ;
#39933=EDGE_LOOP ( 'NONE', ( #20582, #14162, #40105, #37738 ) ) ;
#39938=EDGE_CURVE ( 'NONE', #12019, #13947, #35170, .T. ) ;
#39947=CARTESIAN_POINT ( 'NONE',  ( -728.8365100919714905, 260.0000000000001705, -199.9999999999890861 ) ) ;
#39954=DIRECTION ( 'NONE',  ( 0.000000000000000000, 0.000000000000000000, 1.000000000000000000 ) ) ;
#39960=EDGE_CURVE ( 'NONE', #18073, #21723, #27505, .T. ) ;
#39984=ADVANCED_FACE ( 'NONE', ( #30515 ), #12982, .F. ) ;
#39986=DIRECTION ( 'NONE',  ( 0.000000000000000000, 0.000000000000000000, 1.000000000000000000 ) ) ;
#40012=VERTEX_POINT ( 'NONE', #34675 ) ;
#40049=CARTESIAN_POINT ( 'NONE',  ( 181.1634899080285948, 256.5000000000000000, -197.2499999999955094 ) ) ;
#40050=LINE ( 'NONE', #19245, #41746 ) ;
#40083=DIRECTION ( 'NONE',  ( -0.000000000000000000, 1.000000000000000000, -0.000000000000000000 ) ) ;
#40105=ORIENTED_EDGE ( 'NONE', *, *, #28933, .F. ) ;
#40112=VECTOR ( 'NONE', #1821, 1000.000000000000114 ) ;
#40153=EDGE_LOOP ( 'NONE', ( #37550, #35919, #27784, #38938 ) ) ;
#40186=CIRCLE ( 'NONE', #26876, 6.119000000000013095 ) ;
#40192=VECTOR ( 'NONE', #19143, 1000.000000000000000 ) ;
#40196=LINE ( 'NONE', #2060, #40112 ) ;
#40201=ORIENTED_EDGE ( 'NONE', *, *, #9440, .T. ) ;
#40220=ADVANCED_FACE ( 'NONE', ( #7417, #32120 ), #14116, .F. ) ;
#40230=AXIS2_PLACEMENT_3D ( 'NONE', #13295, #20660, #13068 ) ;
#40245=VERTEX_POINT ( 'NONE', #714 ) ;
#40248=EDGE_CURVE ( 'NONE', #13947, #30459, #28189, .T. ) ;
#40262=FACE_OUTER_BOUND ( 'NONE', #3439, .T. ) ;
#40298=UNCERTAINTY_MEASURE_WITH_UNIT (LENGTH_MEASURE( 1.000000000000000082E-05 ), #17635, 'distance_accuracy_value', 'NONE');
#40304=ADVANCED_FACE ( 'NONE', ( #24723 ), #32582, .F. ) ;
#40312=VERTEX_POINT ( 'NONE', #11105 ) ;
#40317=CYLINDRICAL_SURFACE ( 'NONE', #15223, 6.119000000000013095 ) ;
#40318=LINE ( 'NONE', #36613, #11537 ) ;
#40322=CARTESIAN_POINT ( 'NONE',  ( 571.1634899080285095, 239.9999999999999432, -202.7499999999980105 ) ) ;
#40326=DIRECTION ( 'NONE',  ( -0.000000000000000000, 1.000000000000000000, -0.000000000000000000 ) ) ;
#40332=FACE_BOUND ( 'NONE', #32906, .T. ) ;
#40345=CARTESIAN_POINT ( 'NONE',  ( 181.1634899080285948, 260.0000000000000000, -199.9999999999953957 ) ) ;
#40363=AXIS2_PLACEMENT_3D ( 'NONE', #2704, #33657, #37574 ) ;
#40389=ORIENTED_EDGE ( 'NONE', *, *, #35177, .T. ) ;
#40425=CIRCLE ( 'NONE', #30087, 2.749999999999863665 ) ;
#40439=CARTESIAN_POINT ( 'NONE',  ( -728.8365100919714905, 260.0000000000001705, -202.7499999999889440 ) ) ;
#40478=EDGE_CURVE ( 'NONE', #22607, #10815, #24848, .T. ) ;
#40483=VERTEX_POINT ( 'NONE', #21268 ) ;
#40506=DIRECTION ( 'NONE',  ( -0.000000000000000000, 1.000000000000000000, -0.000000000000000000 ) ) ;
#40519=VERTEX_POINT ( 'NONE', #4192 ) ;
#40531=DIRECTION ( 'NONE',  ( -0.000000000000000000, 1.000000000000000000, -0.000000000000000000 ) ) ;
#40533=EDGE_LOOP ( 'NONE', ( #29898, #30908, #41646, #26908 ) ) ;
#40535=DIRECTION ( 'NONE',  ( -0.000000000000000000, 1.000000000000000000, -0.000000000000000000 ) ) ;
#40544=CARTESIAN_POINT ( 'NONE',  ( -468.8365100919714337, 258.0940000000001646, -199.9999999999908766 ) ) ;
#40551=CIRCLE ( 'NONE', #7352, 2.749999999999919176 ) ;
#40594=CYLINDRICAL_SURFACE ( 'NONE', #18969, 2.749999999999835687 ) ;
#40600=EDGE_LOOP ( 'NONE', ( #6770, #10506, #31376, #19888 ) ) ;
#40603=DIRECTION ( 'NONE',  ( -1.000000000000000000, 0.000000000000000000, 0.000000000000000000 ) ) ;
#40682=ORIENTED_EDGE ( 'NONE', *, *, #17337, .T. ) ;
#40686=ORIENTED_EDGE ( 'NONE', *, *, #16475, .F. ) ;
#40695=EDGE_CURVE ( 'NONE', #34711, #12298, #40196, .T. ) ;
#40716=CARTESIAN_POINT ( 'NONE',  ( -208.8365100919714052, 260.0000000000001137, -199.9999999999926956 ) ) ;
#40725=CARTESIAN_POINT ( 'NONE',  ( 181.1634899080285948, 260.0000000000000000, -197.2499999999955662 ) ) ;
#40739=PLANE ( 'NONE',  #14457 ) ;
#40740=FACE_OUTER_BOUND ( 'NONE', #19707, .T. ) ;
#40748=DIRECTION ( 'NONE',  ( 0.000000000000000000, 0.000000000000000000, 1.000000000000000000 ) ) ;
#40754=CARTESIAN_POINT ( 'NONE',  ( 571.1634899080285095, 259.9999999999999432, -208.0249999999981014 ) ) ;
#40763=DIRECTION ( 'NONE',  ( -0.000000000000000000, 1.000000000000000000, -0.000000000000000000 ) ) ;
#40770=LINE ( 'NONE', #29922, #15820 ) ;
#40778=EDGE_CURVE ( 'NONE', #34351, #26697, #31987, .T. ) ;
#40782=ADVANCED_FACE ( 'NONE', ( #8113 ), #26083, .F. ) ;
#40792=AXIS2_PLACEMENT_3D ( 'NONE', #17243, #28789, #10778 ) ;
#40802=CARTESIAN_POINT ( 'NONE',  ( 311.1634899080286232, 260.0000000000000000, -193.8809999999963338 ) ) ;
#40829=VERTEX_POINT ( 'NONE', #33258 ) ;
#40839=DIRECTION ( 'NONE',  ( -0.000000000000000000, 1.000000000000000000, -0.000000000000000000 ) ) ;
#40850=EDGE_CURVE ( 'NONE', #30459, #9099, #13540, .T. ) ;
#40865=PLANE ( 'NONE',  #41050 ) ;
#40867=DIRECTION ( 'NONE',  ( -0.000000000000000000, 1.000000000000000000, -0.000000000000000000 ) ) ;
#40906=EDGE_LOOP ( 'NONE', ( #6861, #42849 ) ) ;
#40922=CARTESIAN_POINT ( 'NONE',  ( 311.1634899080286232, 260.0000000000000000, -191.9749999999963279 ) ) ;
#40932=CARTESIAN_POINT ( 'NONE',  ( -338.8365100919713200, 256.5000000000001137, -199.9999999999917861 ) ) ;
#40942=DIRECTION ( 'NONE',  ( -0.000000000000000000, 1.000000000000000000, -0.000000000000000000 ) ) ;
#40963=VERTEX_POINT ( 'NONE', #16853 ) ;
#40978=CIRCLE ( 'NONE', #3373, 8.025000000000003908 ) ;
#40980=ORIENTED_EDGE ( 'NONE', *, *, #26084, .F. ) ;
#40996=DIRECTION ( 'NONE',  ( -0.000000000000000000, 1.000000000000000000, -0.000000000000000000 ) ) ;
#41007=DIRECTION ( 'NONE',  ( 0.000000000000000000, 0.000000000000000000, 1.000000000000000000 ) ) ;
#41017=EDGE_CURVE ( 'NONE', #8247, #16583, #15023, .T. ) ;
#41023=ORIENTED_EDGE ( 'NONE', *, *, #17520, .T. ) ;
#41029=ORIENTED_EDGE ( 'NONE', *, *, #36014, .T. ) ;
#41041=ADVANCED_FACE ( 'NONE', ( #9229 ), #13158, .F. ) ;
#41043=CARTESIAN_POINT ( 'NONE',  ( -78.83651009197140525, 256.5000000000000568, -199.9999999999936051 ) ) ;
#41050=AXIS2_PLACEMENT_3D ( 'NONE', #2755, #43861, #27919 ) ;
#41056=CARTESIAN_POINT ( 'NONE',  ( -858.8365100919713768, 260.0000000000002274, -191.9749999999881993 ) ) ;
#41070=VECTOR ( 'NONE', #42421, 1000.000000000000000 ) ;
#41120=VECTOR ( 'NONE', #40326, 1000.000000000000000 ) ;
#41128=LINE ( 'NONE', #15952, #3636 ) ;
#41132=EDGE_CURVE ( 'NONE', #18880, #25919, #43749, .T. ) ;
#41149=CIRCLE ( 'NONE', #16080, 6.119000000000013095 ) ;
#41155=ORIENTED_EDGE ( 'NONE', *, *, #15105, .F. ) ;
#41176=DIRECTION ( 'NONE',  ( 0.000000000000000000, 0.000000000000000000, 1.000000000000000000 ) ) ;
#41197=VERTEX_POINT ( 'NONE', #2758 ) ;
#41205=VECTOR ( 'NONE', #44632, 1000.000000000000114 ) ;
#41216=CARTESIAN_POINT ( 'NONE',  ( -879.9999999999992042, 240.0000000000002274, -219.9999999999999716 ) ) ;
#41219=FACE_OUTER_BOUND ( 'NONE', #13344, .T. ) ;
#41223=DIRECTION ( 'NONE',  ( 0.000000000000000000, 0.000000000000000000, 1.000000000000000000 ) ) ;
#41229=DIRECTION ( 'NONE',  ( 0.000000000000000000, 0.000000000000000000, 1.000000000000000000 ) ) ;
#41243=CARTESIAN_POINT ( 'NONE',  ( -468.8365100919714337, 260.0000000000001705, -191.9749999999908709 ) ) ;
#41246=VERTEX_POINT ( 'NONE', #45244 ) ;
#41250=FACE_OUTER_BOUND ( 'NONE', #32286, .T. ) ;
#41260=VERTEX_POINT ( 'NONE', #34838 ) ;
#41273=CONICAL_SURFACE ( 'NONE', #16942, 8.025000000000003908, 0.7853981633974482790 ) ;
#41276=DIRECTION ( 'NONE',  ( -0.000000000000000000, 1.000000000000000000, -0.000000000000000000 ) ) ;
#41312=CARTESIAN_POINT ( 'NONE',  ( 571.1634899080285095, 259.9999999999999432, -199.9999999999981526 ) ) ;
#41326=CARTESIAN_POINT ( 'NONE',  ( -208.8365100919714052, 258.0940000000001078, -206.1189999999926954 ) ) ;
#41329=DIRECTION ( 'NONE',  ( 0.000000000000000000, 0.000000000000000000, 1.000000000000000000 ) ) ;
#41339=CARTESIAN_POINT ( 'NONE',  ( 181.1634899080285948, 260.0000000000000000, -208.0249999999954014 ) ) ;
#41345=CARTESIAN_POINT ( 'NONE',  ( -468.8365100919714337, 258.0940000000001646, -193.8809999999909053 ) ) ;
#41381=ORIENTED_EDGE ( 'NONE', *, *, #6043, .F. ) ;
#41389=EDGE_LOOP ( 'NONE', ( #42670, #16419, #33562, #41029 ) ) ;
#41395=ADVANCED_FACE ( 'NONE', ( #3898 ), #44451, .F. ) ;
#41429=VERTEX_POINT ( 'NONE', #11061 ) ;
#41436=ORIENTED_EDGE ( 'NONE', *, *, #31148, .T. ) ;
#41503=DIRECTION ( 'NONE',  ( 1.892425610156518354E-16, 1.000000000000000000, -0.000000000000000000 ) ) ;
#41524=ORIENTED_EDGE ( 'NONE', *, *, #39356, .T. ) ;
#41534=ADVANCED_FACE ( 'NONE', ( #42918, #14765 ), #28838, .F. ) ;
#41538=EDGE_CURVE ( 'NONE', #2952, #40312, #11284, .T. ) ;
#41548=DIRECTION ( 'NONE',  ( 0.000000000000000000, 0.000000000000000000, 1.000000000000000000 ) ) ;
#41590=CIRCLE ( 'NONE', #43075, 6.118999999999985562 ) ;
#41607=EDGE_LOOP ( 'NONE', ( #36258, #9343 ) ) ;
#41626=DIRECTION ( 'NONE',  ( -0.000000000000000000, 1.000000000000000000, -0.000000000000000000 ) ) ;
#41646=ORIENTED_EDGE ( 'NONE', *, *, #33669, .T. ) ;
#41663=AXIS2_PLACEMENT_3D ( 'NONE', #43268, #39359, #7489 ) ;
#41666=DIRECTION ( 'NONE',  ( 0.000000000000000000, 0.000000000000000000, 1.000000000000000000 ) ) ;
#41667=EDGE_LOOP ( 'NONE', ( #42678, #22538 ) ) ;
#41679=LINE ( 'NONE', #13499, #45166 ) ;
#41683=AXIS2_PLACEMENT_3D ( 'NONE', #16114, #30199, #35832 ) ;
#41697=AXIS2_PLACEMENT_3D ( 'NONE', #30723, #32545, #215 ) ;
#41702=EDGE_CURVE ( 'NONE', #10586, #32983, #24526, .T. ) ;
#41736=DIRECTION ( 'NONE',  ( 0.000000000000000000, 0.000000000000000000, 1.000000000000000000 ) ) ;
#41740=CARTESIAN_POINT ( 'NONE',  ( 831.1634899080286232, 259.9999999999998863, -208.0249999999998920 ) ) ;
#41746=VECTOR ( 'NONE', #12544, 1000.000000000000000 ) ;
#41751=PRODUCT_DEFINITION_SHAPE ( 'NONE', 'NONE',  #33777 ) ;
#41768=ORIENTED_EDGE ( 'NONE', *, *, #1284, .F. ) ;
#41810=AXIS2_PLACEMENT_3D ( 'NONE', #14345, #249, #18039 ) ;
#41830=ORIENTED_EDGE ( 'NONE', *, *, #16234, .F. ) ;
#41843=DIRECTION ( 'NONE',  ( -0.000000000000000000, 1.000000000000000000, -0.000000000000000000 ) ) ;
#41855=EDGE_CURVE ( 'NONE', #32983, #12347, #22574, .T. ) ;
#41866=CYLINDRICAL_SURFACE ( 'NONE', #7041, 6.118999999999985562 ) ;
#41873=AXIS2_PLACEMENT_3D ( 'NONE', #28759, #25513, #14682 ) ;
#41901=ORIENTED_EDGE ( 'NONE', *, *, #2759, .F. ) ;
#41925=ADVANCED_FACE ( 'NONE', ( #14983 ), #44049, .F. ) ;
#41931=FACE_BOUND ( 'NONE', #13827, .T. ) ;
#41958=DIRECTION ( 'NONE',  ( -0.000000000000000000, 1.000000000000000000, -0.000000000000000000 ) ) ;
#41964=ADVANCED_FACE ( 'NONE', ( #37110 ), #26735, .F. ) ;
#41966=DIRECTION ( 'NONE',  ( 0.000000000000000000, 0.000000000000000000, 1.000000000000000000 ) ) ;
#41973=FACE_OUTER_BOUND ( 'NONE', #9737, .T. ) ;
#41999=CARTESIAN_POINT ( 'NONE',  ( -728.8365100919714905, 240.0000000000001990, -202.7499999999889440 ) ) ;
#42002=AXIS2_PLACEMENT_3D ( 'NONE', #2534, #37646, #20088 ) ;
#42017=CARTESIAN_POINT ( 'NONE',  ( 707.2824899080285377, 256.4999999999999432, -199.9999999999990337 ) ) ;
#42029=DIRECTION ( 'NONE',  ( -0.000000000000000000, 1.000000000000000000, -0.000000000000000000 ) ) ;
#42044=ORIENTED_EDGE ( 'NONE', *, *, #7550, .F. ) ;
#42049=DIRECTION ( 'NONE',  ( 0.000000000000000000, 0.000000000000000000, 1.000000000000000000 ) ) ;
#42062=DIRECTION ( 'NONE',  ( -0.000000000000000000, 1.000000000000000000, -0.000000000000000000 ) ) ;
#42077=CARTESIAN_POINT ( 'NONE',  ( 831.1634899080286232, 259.9999999999998863, -191.9749999999999943 ) ) ;
#42102=ORIENTED_EDGE ( 'NONE', *, *, #42169, .F. ) ;
#42155=ORIENTED_EDGE ( 'NONE', *, *, #22701, .T. ) ;
#42169=EDGE_CURVE ( 'NONE', #5383, #38472, #42972, .T. ) ;
#42190=CARTESIAN_POINT ( 'NONE',  ( 441.1634899080286232, 239.9999999999999716, -202.7499999999971010 ) ) ;
#42191=DIRECTION ( 'NONE',  ( -0.000000000000000000, 1.000000000000000000, -0.000000000000000000 ) ) ;
#42217=AXIS2_PLACEMENT_3D ( 'NONE', #18908, #22803, #32761 ) ;
#42233=CARTESIAN_POINT ( 'NONE',  ( -879.9999999999992042, 240.0000000000002274, -219.9999999999999716 ) ) ;
#42236=CARTESIAN_POINT ( 'NONE',  ( 879.9999999999992042, 239.9999999999998863, -179.9999999999999716 ) ) ;
#42269=ORIENTED_EDGE ( 'NONE', *, *, #19866, .T. ) ;
#42282=CARTESIAN_POINT ( 'NONE',  ( 317.2824899080285945, 256.5000000000000000, -199.9999999999963336 ) ) ;
#42304=CARTESIAN_POINT ( 'NONE',  ( 311.1634899080286232, 260.0000000000000000, -199.9999999999963336 ) ) ;
#42311=FACE_OUTER_BOUND ( 'NONE', #43736, .T. ) ;
#42324=VECTOR ( 'NONE', #23636, 1000.000000000000000 ) ;
#42338=DIRECTION ( 'NONE',  ( -0.000000000000000000, 1.000000000000000000, -0.000000000000000000 ) ) ;
#42341=VERTEX_POINT ( 'NONE', #41740 ) ;
#42362=CARTESIAN_POINT ( 'NONE',  ( 831.1634899080286232, 259.9999999999998863, -202.7499999999998295 ) ) ;
#42394=FACE_OUTER_BOUND ( 'NONE', #16123, .T. ) ;
#42403=FACE_OUTER_BOUND ( 'NONE', #2573, .T. ) ;
#42421=DIRECTION ( 'NONE',  ( 0.000000000000000000, 0.7071067811865526798, 0.7071067811865423547 ) ) ;
#42426=CIRCLE ( 'NONE', #13678, 6.118999999999985562 ) ;
#42430=EDGE_LOOP ( 'NONE', ( #27794, #9561 ) ) ;
#42446=ORIENTED_EDGE ( 'NONE', *, *, #28109, .T. ) ;
#42463=PLANE ( 'NONE',  #44750 ) ;
#42501=VECTOR ( 'NONE', #20175, 1000.000000000000000 ) ;
#42507=VERTEX_POINT ( 'NONE', #18178 ) ;
#42532=ADVANCED_FACE ( 'NONE', ( #28560, #41973 ), #42867, .F. ) ;
#42537=EDGE_CURVE ( 'NONE', #13600, #25447, #14481, .T. ) ;
#42559=VERTEX_POINT ( 'NONE', #13799 ) ;
#42561=VECTOR ( 'NONE', #42917, 1000.000000000000114 ) ;
#42568=CARTESIAN_POINT ( 'NONE',  ( -728.8365100919714905, 256.5000000000001705, -199.9999999999890861 ) ) ;
#42571=ORIENTED_EDGE ( 'NONE', *, *, #25287, .F. ) ;
#42572=ORIENTED_EDGE ( 'NONE', *, *, #14023, .F. ) ;
#42580=ORIENTED_EDGE ( 'NONE', *, *, #24391, .F. ) ;
#42592=CIRCLE ( 'NONE', #30775, 2.749999999999919176 ) ;
#42614=FACE_OUTER_BOUND ( 'NONE', #8598, .T. ) ;
#42622=CARTESIAN_POINT ( 'NONE',  ( -468.8365100919714337, 240.0000000000001421, -197.2499999999910187 ) ) ;
#42639=PLANE ( 'NONE',  #5580 ) ;
#42661=CARTESIAN_POINT ( 'NONE',  ( -208.8365100919714052, 260.0000000000001137, -191.9749999999926899 ) ) ;
#42670=ORIENTED_EDGE ( 'NONE', *, *, #36816, .F. ) ;
#42674=VERTEX_POINT ( 'NONE', #150 ) ;
#42678=ORIENTED_EDGE ( 'NONE', *, *, #17953, .T. ) ;
#42696=CARTESIAN_POINT ( 'NONE',  ( -858.8365100919713768, 260.0000000000002274, -199.9999999999881481 ) ) ;
#42704=DIRECTION ( 'NONE',  ( 0.000000000000000000, 0.000000000000000000, 1.000000000000000000 ) ) ;
#42720=CIRCLE ( 'NONE', #2155, 6.118999999999985562 ) ;
#42741=EDGE_CURVE ( 'NONE', #33435, #7627, #9069, .T. ) ;
#42760=EDGE_CURVE ( 'NONE', #7627, #33435, #12021, .T. ) ;
#42794=ORIENTED_EDGE ( 'NONE', *, *, #6120, .T. ) ;
#42798=ORIENTED_EDGE ( 'NONE', *, *, #33183, .F. ) ;
#42807=CYLINDRICAL_SURFACE ( 'NONE', #39537, 2.749999999999863665 ) ;
#42814=PLANE ( 'NONE',  #39301 ) ;
#42826=CYLINDRICAL_SURFACE ( 'NONE', #35007, 6.118999999999985562 ) ;
#42835=ORIENTED_EDGE ( 'NONE', *, *, #40478, .T. ) ;
#42849=ORIENTED_EDGE ( 'NONE', *, *, #8063, .T. ) ;
#42854=FACE_BOUND ( 'NONE', #12965, .T. ) ;
#42858=DIRECTION ( 'NONE',  ( -0.000000000000000000, 1.000000000000000000, -0.000000000000000000 ) ) ;
#42867=PLANE ( 'NONE',  #40792 ) ;
#42885=ORIENTED_EDGE ( 'NONE', *, *, #40778, .T. ) ;
#42896=EDGE_CURVE ( 'NONE', #11829, #38048, #36626, .T. ) ;
#42917=DIRECTION ( 'NONE',  ( 0.000000000000000000, 0.7071067811865474617, 0.7071067811865474617 ) ) ;
#42918=FACE_BOUND ( 'NONE', #8485, .T. ) ;
#42925=FACE_OUTER_BOUND ( 'NONE', #31617, .T. ) ;
#42950=DIRECTION ( 'NONE',  ( 0.000000000000000000, 0.000000000000000000, 1.000000000000000000 ) ) ;
#42963=DIRECTION ( 'NONE',  ( -0.000000000000000000, 1.000000000000000000, -0.000000000000000000 ) ) ;
#42972=CIRCLE ( 'NONE', #11987, 2.749999999999919176 ) ;
#42984=DIRECTION ( 'NONE',  ( 0.000000000000000000, 0.000000000000000000, 1.000000000000000000 ) ) ;
#43001=ORIENTED_EDGE ( 'NONE', *, *, #9484, .F. ) ;
#43003=ADVANCED_FACE ( 'NONE', ( #11907, #40332, #29907, #832, #29251, #14931, #8446, #1054, #22077, #43097, #22749, #11463, #5194, #33162, #33368 ), #7771, .T. ) ;
#43019=EDGE_CURVE ( 'NONE', #45067, #8740, #18683, .T. ) ;
#43044=AXIS2_PLACEMENT_3D ( 'NONE', #20296, #27237, #41329 ) ;
#43051=EDGE_CURVE ( 'NONE', #44542, #30554, #22318, .T. ) ;
#43063=PRODUCT_DEFINITION_CONTEXT ( 'detailed design', #16367, 'design' ) ;
#43075=AXIS2_PLACEMENT_3D ( 'NONE', #20197, #40763, #43999 ) ;
#43083=CARTESIAN_POINT ( 'NONE',  ( 311.1634899080286232, 256.5000000000000000, -206.1189999999963050 ) ) ;
#43094=DIRECTION ( 'NONE',  ( 0.000000000000000000, 0.000000000000000000, 1.000000000000000000 ) ) ;
#43097=FACE_BOUND ( 'NONE', #13211, .T. ) ;
#43103=EDGE_CURVE ( 'NONE', #15531, #14461, #20421, .T. ) ;
#43108=CARTESIAN_POINT ( 'NONE',  ( 441.1634899080286232, 256.4999999999999432, -199.9999999999972431 ) ) ;
#43110=EDGE_CURVE ( 'NONE', #34351, #16943, #34516, .T. ) ;
#43147=STYLED_ITEM('',(#45779),#2718);
#43168=DIRECTION ( 'NONE',  ( 0.000000000000000000, 0.000000000000000000, 1.000000000000000000 ) ) ;
#43177=DIRECTION ( 'NONE',  ( -0.000000000000000000, 1.000000000000000000, -0.000000000000000000 ) ) ;
#43181=ORIENTED_EDGE ( 'NONE', *, *, #43367, .F. ) ;
#43198=FACE_OUTER_BOUND ( 'NONE', #35039, .T. ) ;
#43239=DIRECTION ( 'NONE',  ( 0.000000000000000000, 0.000000000000000000, 1.000000000000000000 ) ) ;
#43257=CONICAL_SURFACE ( 'NONE', #16685, 8.024999999999948841, 0.7853981633974337351 ) ;
#43265=CARTESIAN_POINT ( 'NONE',  ( 441.1634899080286232, 259.9999999999999432, -199.9999999999972431 ) ) ;
#43267=EDGE_CURVE ( 'NONE', #31071, #8149, #31198, .T. ) ;
#43268=CARTESIAN_POINT ( 'NONE',  ( 831.1634899080286232, 259.9999999999998863, -199.9999999999999432 ) ) ;
#43273=AXIS2_PLACEMENT_3D ( 'NONE', #9045, #32868, #24666 ) ;
#43279=CARTESIAN_POINT ( 'NONE',  ( 181.1634899080285948, 260.0000000000000000, -191.9749999999953900 ) ) ;
#43298=ORIENTED_EDGE ( 'NONE', *, *, #26419, .F. ) ;
#43306=ORIENTED_EDGE ( 'NONE', *, *, #33916, .F. ) ;
#43316=EDGE_LOOP ( 'NONE', ( #10922, #17582 ) ) ;
#43318=CARTESIAN_POINT ( 'NONE',  ( 51.16348990802859475, 260.0000000000000568, -197.2499999999946851 ) ) ;
#43321=CIRCLE ( 'NONE', #41873, 2.749999999999919176 ) ;
#43323=FACE_OUTER_BOUND ( 'NONE', #37544, .T. ) ;
#43328=DIRECTION ( 'NONE',  ( -0.000000000000000000, 1.000000000000000000, -0.000000000000000000 ) ) ;
#43346=DIRECTION ( 'NONE',  ( 0.000000000000000000, 0.000000000000000000, 1.000000000000000000 ) ) ;
#43357=AXIS2_PLACEMENT_3D ( 'NONE', #4892, #30269, #12499 ) ;
#43367=EDGE_CURVE ( 'NONE', #38472, #5383, #32698, .T. ) ;
#43401=CARTESIAN_POINT ( 'NONE',  ( 311.1634899080286232, 256.5000000000000000, -199.9999999999963336 ) ) ;
#43430=ORIENTED_EDGE ( 'NONE', *, *, #24477, .F. ) ;
#43462=ORIENTED_EDGE ( 'NONE', *, *, #9440, .F. ) ;
#43476=CARTESIAN_POINT ( 'NONE',  ( -338.8365100919713200, 258.0940000000001078, -193.8809999999918148 ) ) ;
#43489=DIRECTION ( 'NONE',  ( -0.000000000000000000, 1.000000000000000000, -0.000000000000000000 ) ) ;
#43491=CARTESIAN_POINT ( 'NONE',  ( 311.1634899080286232, 256.5000000000000000, -199.9999999999963336 ) ) ;
#43497=DIRECTION ( 'NONE',  ( 0.000000000000000000, -0.000000000000000000, -1.000000000000000000 ) ) ;
#43518=EDGE_CURVE ( 'NONE', #40312, #16670, #20863, .T. ) ;
#43570=ADVANCED_FACE ( 'NONE', ( #38216 ), #31947, .F. ) ;
#43586=DIRECTION ( 'NONE',  ( 0.000000000000000000, 0.000000000000000000, 1.000000000000000000 ) ) ;
#43631=ORIENTED_EDGE ( 'NONE', *, *, #90, .T. ) ;
#43657=DIRECTION ( 'NONE',  ( 0.000000000000000000, 0.000000000000000000, 1.000000000000000000 ) ) ;
#43663=DIRECTION ( 'NONE',  ( 0.000000000000000000, 0.000000000000000000, 1.000000000000000000 ) ) ;
#43704=LINE ( 'NONE', #29413, #39411 ) ;
#43716=DIRECTION ( 'NONE',  ( 0.000000000000000000, -1.000000000000000000, 0.000000000000000000 ) ) ;
#43729=CARTESIAN_POINT ( 'NONE',  ( -468.8365100919714337, 260.0000000000001705, -193.8809999999909053 ) ) ;
#43736=EDGE_LOOP ( 'NONE', ( #15149, #8000, #20609, #22996 ) ) ;
#43742=DIRECTION ( 'NONE',  ( 0.000000000000000000, 0.000000000000000000, 1.000000000000000000 ) ) ;
#43749=CIRCLE ( 'NONE', #43044, 6.118999999999985562 ) ;
#43754=CARTESIAN_POINT ( 'NONE',  ( 571.1634899080285095, 259.9999999999999432, -199.9999999999981526 ) ) ;
#43780=CIRCLE ( 'NONE', #31266, 2.749999999999863665 ) ;
#43826=CARTESIAN_POINT ( 'NONE',  ( -78.83651009197140525, 260.0000000000000568, -199.9999999999936051 ) ) ;
#43842=PLANE ( 'NONE',  #31310 ) ;
#43861=DIRECTION ( 'NONE',  ( -0.000000000000000000, 0.000000000000000000, 1.000000000000000000 ) ) ;
#43876=DIRECTION ( 'NONE',  ( -0.000000000000000000, 1.000000000000000000, -0.000000000000000000 ) ) ;
#43880=AXIS2_PLACEMENT_3D ( 'NONE', #34220, #1671, #15776 ) ;
#43895=DIRECTION ( 'NONE',  ( -0.000000000000000000, 1.000000000000000000, -0.000000000000000000 ) ) ;
#43896=AXIS2_PLACEMENT_3D ( 'NONE', #31740, #335, #39376 ) ;
#43969=VECTOR ( 'NONE', #36721, 1000.000000000000000 ) ;
#43985=AXIS2_PLACEMENT_3D ( 'NONE', #37216, #36991, #1437 ) ;
#43994=VECTOR ( 'NONE', #9572, 1000.000000000000000 ) ;
#43999=DIRECTION ( 'NONE',  ( 0.000000000000000000, 0.000000000000000000, 1.000000000000000000 ) ) ;
#44006=AXIS2_PLACEMENT_3D ( 'NONE', #33419, #44744, #9403 ) ;
#44007=DIRECTION ( 'NONE',  ( 0.000000000000000000, 0.000000000000000000, 1.000000000000000000 ) ) ;
#44011=CARTESIAN_POINT ( 'NONE',  ( -598.8365100919716042, 260.0000000000001705, -199.9999999999899671 ) ) ;
#44027=VERTEX_POINT ( 'NONE', #41056 ) ;
#44042=EDGE_CURVE ( 'NONE', #2736, #17707, #29034, .T. ) ;
#44045=DIRECTION ( 'NONE',  ( 0.000000000000000000, 0.000000000000000000, 1.000000000000000000 ) ) ;
#44048=DIRECTION ( 'NONE',  ( -0.000000000000000000, 1.000000000000000000, -0.000000000000000000 ) ) ;
#44049=CYLINDRICAL_SURFACE ( 'NONE', #2371, 6.119000000000013095 ) ;
#44070=ORIENTED_EDGE ( 'NONE', *, *, #20206, .T. ) ;
#44076=ORIENTED_EDGE ( 'NONE', *, *, #26922, .F. ) ;
#44100=DIRECTION ( 'NONE',  ( -0.000000000000000000, 1.000000000000000000, -0.000000000000000000 ) ) ;
#44115=CARTESIAN_POINT ( 'NONE',  ( 831.1634899080286232, 258.0939999999998804, -199.9999999999999432 ) ) ;
#44148=EDGE_LOOP ( 'NONE', ( #16803, #21328 ) ) ;
#44152=CARTESIAN_POINT ( 'NONE',  ( 51.16348990802859475, 240.0000000000000568, -202.7499999999943441 ) ) ;
#44155=EDGE_LOOP ( 'NONE', ( #12554, #2021 ) ) ;
#44157=ADVANCED_FACE ( 'NONE', ( #33666 ), #2469, .F. ) ;
#44186=ADVANCED_FACE ( 'NONE', ( #34793 ), #6409, .F. ) ;
#44211=ORIENTED_EDGE ( 'NONE', *, *, #13072, .T. ) ;
#44230=FACE_OUTER_BOUND ( 'NONE', #5714, .T. ) ;
#44261=ORIENTED_EDGE ( 'NONE', *, *, #19848, .F. ) ;
#44297=LINE ( 'NONE', #5052, #40192 ) ;
#44342=DIRECTION ( 'NONE',  ( -0.000000000000000000, 1.000000000000000000, -0.000000000000000000 ) ) ;
#44343=CARTESIAN_POINT ( 'NONE',  ( -728.8365100919714905, 256.5000000000001705, -206.1189999999890574 ) ) ;
#44353=CARTESIAN_POINT ( 'NONE',  ( 181.1634899080285948, 240.0000000000000284, -199.9999999999953957 ) ) ;
#44361=CIRCLE ( 'NONE', #24443, 8.025000000000003908 ) ;
#44406=CARTESIAN_POINT ( 'NONE',  ( 879.9999999999992042, 239.9999999999998863, -219.9999999999999716 ) ) ;
#44415=DIRECTION ( 'NONE',  ( -0.000000000000000000, 1.000000000000000000, -0.000000000000000000 ) ) ;
#44417=ORIENTED_EDGE ( 'NONE', *, *, #16680, .T. ) ;
#44420=ORIENTED_EDGE ( 'NONE', *, *, #29254, .T. ) ;
#44430=CARTESIAN_POINT ( 'NONE',  ( -468.8365100919714337, 260.0000000000001705, -199.9999999999908766 ) ) ;
#44432=CYLINDRICAL_SURFACE ( 'NONE', #30214, 6.118999999999985562 ) ;
#44433=ORIENTED_EDGE ( 'NONE', *, *, #15984, .T. ) ;
#44444=DIRECTION ( 'NONE',  ( 0.000000000000000000, 0.000000000000000000, 1.000000000000000000 ) ) ;
#44447=DIRECTION ( 'NONE',  ( 8.659560562354807133E-17, 0.7071067811865578978, -0.7071067811865372477 ) ) ;
#44451=CONICAL_SURFACE ( 'NONE', #34090, 8.024999999999948841, 0.7853981633974337351 ) ;
#44455=LINE ( 'NONE', #37759, #11466 ) ;
#44463=FACE_OUTER_BOUND ( 'NONE', #2621, .T. ) ;
#44468=DIRECTION ( 'NONE',  ( 0.000000000000000000, 0.000000000000000000, 1.000000000000000000 ) ) ;
#44501=CARTESIAN_POINT ( 'NONE',  ( 311.1634899080286232, 260.0000000000000000, -199.9999999999963336 ) ) ;
#44528=FACE_OUTER_BOUND ( 'NONE', #30853, .T. ) ;
#44533=CARTESIAN_POINT ( 'NONE',  ( 51.16348990802859475, 256.5000000000000568, -199.9999999999945146 ) ) ;
#44542=VERTEX_POINT ( 'NONE', #42190 ) ;
#44552=AXIS2_PLACEMENT_3D ( 'NONE', #13966, #7033, #37993 ) ;
#44578=CARTESIAN_POINT ( 'NONE',  ( 701.1634899080286232, 239.9999999999999147, -197.2499999999991758 ) ) ;
#44600=EDGE_LOOP ( 'NONE', ( #30674, #36004, #4663, #43631 ) ) ;
#44632=DIRECTION ( 'NONE',  ( 8.659560562354932858E-17, 0.7071067811865474617, -0.7071067811865474617 ) ) ;
#44636=AXIS2_PLACEMENT_3D ( 'NONE', #12332, #40506, #15780 ) ;
#44655=ORIENTED_EDGE ( 'NONE', *, *, #7791, .T. ) ;
#44672=CARTESIAN_POINT ( 'NONE',  ( 571.1634899080285095, 239.9999999999999432, -199.9999999999981526 ) ) ;
#44690=CARTESIAN_POINT ( 'NONE',  ( -598.8365100919716042, 260.0000000000001705, -193.8809999999899674 ) ) ;
#44744=DIRECTION ( 'NONE',  ( -0.000000000000000000, 1.000000000000000000, -0.000000000000000000 ) ) ;
#44750=AXIS2_PLACEMENT_3D ( 'NONE', #38095, #31144, #16850 ) ;
#44778=ORIENTED_EDGE ( 'NONE', *, *, #15389, .F. ) ;
#44780=ADVANCED_FACE ( 'NONE', ( #17943 ), #31984, .F. ) ;
#44811=DIRECTION ( 'NONE',  ( -0.000000000000000000, 1.000000000000000000, -0.000000000000000000 ) ) ;
#44837=ORIENTED_EDGE ( 'NONE', *, *, #5410, .F. ) ;
#44840=CIRCLE ( 'NONE', #26395, 2.749999999999919176 ) ;
#44849=VERTEX_POINT ( 'NONE', #21403 ) ;
#44882=ORIENTED_EDGE ( 'NONE', *, *, #43518, .T. ) ;
#44917=LINE ( 'NONE', #31042, #36327 ) ;
#44918=CARTESIAN_POINT ( 'NONE',  ( -879.9999999999992042, 240.0000000000002274, -179.9999999999999716 ) ) ;
#44971=CARTESIAN_POINT ( 'NONE',  ( -858.8365100919713768, 256.5000000000002274, -199.9999999999881481 ) ) ;
#44972=DIRECTION ( 'NONE',  ( -0.000000000000000000, 1.000000000000000000, -0.000000000000000000 ) ) ;
#44975=LINE ( 'NONE', #36895, #13843 ) ;
#45006=DIRECTION ( 'NONE',  ( -0.000000000000000000, 1.000000000000000000, -0.000000000000000000 ) ) ;
#45009=ORIENTED_EDGE ( 'NONE', *, *, #41702, .F. ) ;
#45024=CARTESIAN_POINT ( 'NONE',  ( -78.83651009197140525, 260.0000000000000568, -199.9999999999936051 ) ) ;
#45047=DIRECTION ( 'NONE',  ( 0.000000000000000000, 0.000000000000000000, 1.000000000000000000 ) ) ;
#45057=ORIENTED_EDGE ( 'NONE', *, *, #10834, .F. ) ;
#45067=VERTEX_POINT ( 'NONE', #23189 ) ;
#45080=DIRECTION ( 'NONE',  ( -0.000000000000000000, 1.000000000000000000, -0.000000000000000000 ) ) ;
#45110=ORIENTED_EDGE ( 'NONE', *, *, #3007, .F. ) ;
#45137=DIRECTION ( 'NONE',  ( -1.000000000000000000, 0.000000000000000000, 0.000000000000000000 ) ) ;
#45166=VECTOR ( 'NONE', #30823, 1000.000000000000000 ) ;
#45167=VECTOR ( 'NONE', #24621, 1000.000000000000000 ) ;
#45204=DIRECTION ( 'NONE',  ( 0.000000000000000000, 0.000000000000000000, 1.000000000000000000 ) ) ;
#45214=EDGE_LOOP ( 'NONE', ( #42571, #33142, #36872, #38525 ) ) ;
#45215=AXIS2_PLACEMENT_3D ( 'NONE', #4981, #22516, #21850 ) ;
#45225=ORIENTED_EDGE ( 'NONE', *, *, #715, .F. ) ;
#45239=VERTEX_POINT ( 'NONE', #26223 ) ;
#45241=DIRECTION ( 'NONE',  ( 1.892425610156518354E-16, 1.000000000000000000, -0.000000000000000000 ) ) ;
#45244=CARTESIAN_POINT ( 'NONE',  ( -598.8365100919716042, 258.0940000000001646, -193.8809999999899674 ) ) ;
#45260=CARTESIAN_POINT ( 'NONE',  ( 571.1634899080285095, 239.9999999999999432, -197.2499999999982947 ) ) ;
#45300=DIRECTION ( 'NONE',  ( 0.000000000000000000, 0.000000000000000000, 1.000000000000000000 ) ) ;
#45331=AXIS2_PLACEMENT_3D ( 'NONE', #470, #910, #42950 ) ;
#45348=SHAPE_REPRESENTATION_RELATIONSHIP ( 'NONE' , 'NONE' ,  #28315, #13364 ) ;
#45355=CIRCLE ( 'NONE', #25429, 6.119000000000013095 ) ;
#45373=LINE ( 'NONE', #34961, #27445 ) ;
#45377=AXIS2_PLACEMENT_3D ( 'NONE', #8891, #16273, #44444 ) ;
#45388=CARTESIAN_POINT ( 'NONE',  ( 831.1634899080286232, 259.9999999999998863, -199.9999999999999432 ) ) ;
#45398=ORIENTED_EDGE ( 'NONE', *, *, #23048, .F. ) ;
#45429=AXIS2_PLACEMENT_3D ( 'NONE', #4062, #28545, #21605 ) ;
#45437=CONICAL_SURFACE ( 'NONE', #11506, 8.025000000000003908, 0.7853981633974428389 ) ;
#45445=AXIS2_PLACEMENT_3D ( 'NONE', #44430, #40531, #8880 ) ;
#45447=LINE ( 'NONE', #13118, #5042 ) ;
#45505=AXIS2_PLACEMENT_3D ( 'NONE', #9514, #41843, #45300 ) ;
#45538=CIRCLE ( 'NONE', #10882, 6.118999999999985562 ) ;
#45563=DIRECTION ( 'NONE',  ( 1.892425610156518354E-16, 1.000000000000000000, -0.000000000000000000 ) ) ;
#45571=CIRCLE ( 'NONE', #2800, 2.749999999999919176 ) ;
#45598=DIRECTION ( 'NONE',  ( 0.000000000000000000, 0.000000000000000000, 1.000000000000000000 ) ) ;
#45658=ORIENTED_EDGE ( 'NONE', *, *, #19344, .T. ) ;
#45714=LINE ( 'NONE', #42233, #37382 ) ;
#45773=COLOUR_RGB('Off White',0.89,0.88,0.83);
#45774=FILL_AREA_STYLE_COLOUR('',#45773);
#45775=FILL_AREA_STYLE('',(#45774));
#45776=SURFACE_STYLE_FILL_AREA(#45775);
#45777=SURFACE_SIDE_STYLE('',(#45776));
#45778=SURFACE_STYLE_USAGE(.BOTH.,#45777);
#45779=PRESENTATION_STYLE_ASSIGNMENT((#45778));
ENDSEC;
END-ISO-10303-21;
